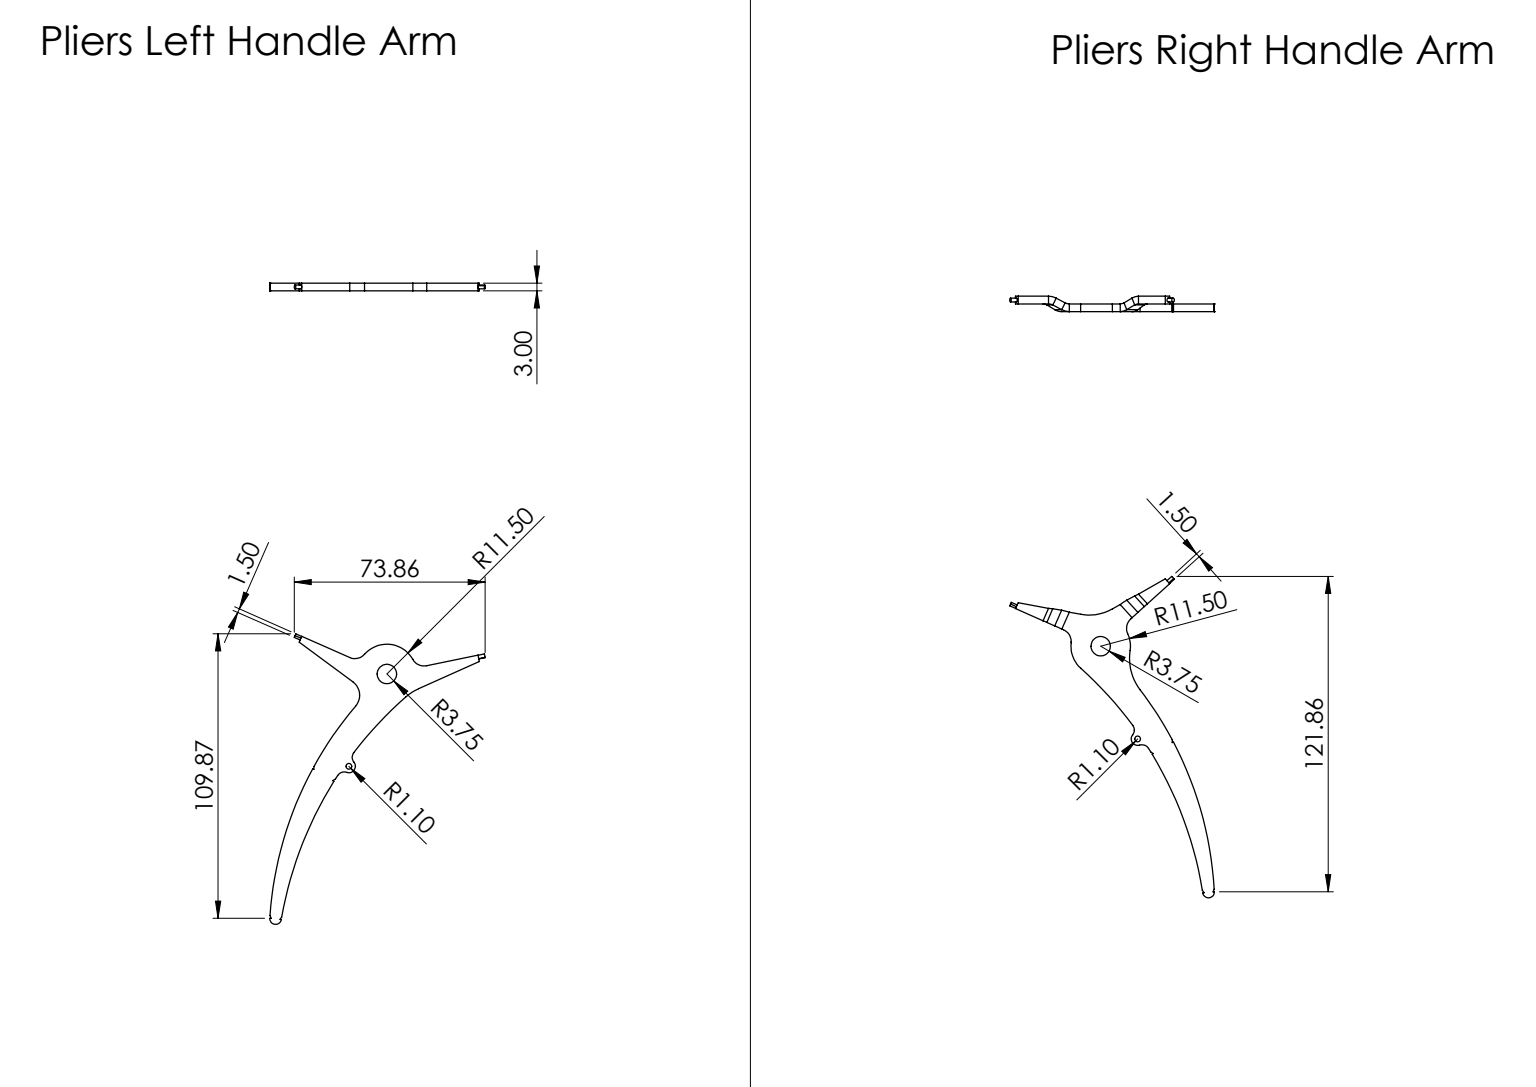
ISO-10303-21;
HEADER;
FILE_DESCRIPTION (('STEP AP214'),
    '1' );
FILE_NAME ('Pliers Left Handle Arm.step',
    '2026-10-09T15:01:35',
    ( '' ),
    ( '' ),
    'SwSTEP 2.0',
    'SolidWorks 2026',
    '' );
FILE_SCHEMA (( 'AUTOMOTIVE_DESIGN' ));
ENDSEC;

DATA;
#3=DIRECTION ( 'NONE',  ( -5.715354789860003484E-18, -9.999836672264337477E-16, 1.000000000000000000 ) ) ;
#4=DIRECTION ( 'NONE',  ( -5.715354789860003484E-18, -9.999836672264337477E-16, 1.000000000000000000 ) ) ;
#12=CARTESIAN_POINT ( 'NONE',  ( 1.714606436958001585E-17, 2.999951001679301835E-15, -3.000000000000000888 ) ) ;
#13=CARTESIAN_POINT ( 'NONE',  ( 37.74350889372263396, 7.597106414893625370, -1.944871132915118705 ) ) ;
#14=CARTESIAN_POINT ( 'NONE',  ( 10.02759472486470926, 5.630039434485818894, -2.999999999999995115 ) ) ;
#21=ORIENTED_EDGE ( 'NONE', *, *, #345, .T. ) ;
#22=ORIENTED_EDGE ( 'NONE', *, *, #4795, .T. ) ;
#27=EDGE_CURVE ( 'NONE', #7442, #6679, #395, .T. ) ;
#42=CYLINDRICAL_SURFACE ( 'NONE', #5055, 2.999999999999999556 ) ;
#44=AXIS2_PLACEMENT_3D ( 'NONE', #1509, #3865, #2736 ) ;
#45=ORIENTED_EDGE ( 'NONE', *, *, #3432, .T. ) ;
#53=CARTESIAN_POINT ( 'NONE',  ( -28.22553731214382111, -35.79092421365019305, -3.595165860846261460E-14 ) ) ;
#55=CARTESIAN_POINT ( 'NONE',  ( -13.19674249314596892, -2.997380612392111843, -3.000000000000003997 ) ) ;
#59=CARTESIAN_POINT ( 'NONE',  ( -14.70408710852078116, -35.66654345889202204, -3.000000000000036415 ) ) ;
#63=DIRECTION ( 'NONE',  ( -5.715354789860003484E-18, -9.999836672264337477E-16, 1.000000000000000000 ) ) ;
#65=ORIENTED_EDGE ( 'NONE', *, *, #2017, .F. ) ;
#74=VERTEX_POINT ( 'NONE', #2232 ) ;
#88=CYLINDRICAL_SURFACE ( 'NONE', #3600, 147.0000000000000284 ) ;
#96=CARTESIAN_POINT ( 'NONE',  ( 30.52077159997833533, 5.488396937353885896, -1.499999999999994893 ) ) ;
#100=DIRECTION ( 'NONE',  ( -0.9999836672264332815, 0.005715354789859956701, 0.000000000000000000 ) ) ;
#112=EDGE_CURVE ( 'NONE', #2053, #3816, #7103, .T. ) ;
#133=FACE_OUTER_BOUND ( 'NONE', #7338, .T. ) ;
#137=ORIENTED_EDGE ( 'NONE', *, *, #2521, .F. ) ;
#142=PLANE ( 'NONE',  #2794 ) ;
#145=CARTESIAN_POINT ( 'NONE',  ( 30.52077159997833533, 5.488396937353885896, -1.499999999999994893 ) ) ;
#155=DIRECTION ( 'NONE',  ( -0.9999836672264332815, 0.005715354789859956701, 0.000000000000000000 ) ) ;
#160=CARTESIAN_POINT ( 'NONE',  ( -28.26642576027046516, -36.90973657692984489, -3.000000000000037748 ) ) ;
#164=AXIS2_PLACEMENT_3D ( 'NONE', #6562, #6008, #5019 ) ;
#168=AXIS2_PLACEMENT_3D ( 'NONE', #4159, #3722, #2491 ) ;
#171=CARTESIAN_POINT ( 'NONE',  ( -16.51707533432788111, -40.85914143033993895, -3.000000000000041744 ) ) ;
#172=ORIENTED_EDGE ( 'NONE', *, *, #3864, .T. ) ;
#173=ORIENTED_EDGE ( 'NONE', *, *, #526, .F. ) ;
#176=CIRCLE ( 'NONE', #6665, 0.7499999999999893419 ) ;
#182=ORIENTED_EDGE ( 'NONE', *, *, #4904, .T. ) ;
#194=DIRECTION ( 'NONE',  ( 9.251858538542970644E-15, 2.775557561562891351E-14, 1.000000000000000000 ) ) ;
#201=DIRECTION ( 'NONE',  ( 0.8552446107963830313, 0.5182245224839744369, 5.231040848230092092E-16 ) ) ;
#211=EDGE_LOOP ( 'NONE', ( #3520, #3050, #137, #3824 ) ) ;
#220=ORIENTED_EDGE ( 'NONE', *, *, #5909, .F. ) ;
#221=DIRECTION ( 'NONE',  ( 0.1200071523045019850, -0.5808948794702039065, -0.8050834878452428622 ) ) ;
#223=DIRECTION ( 'NONE',  ( 0.4039838799357178822, 0.9147661038495488173, -2.999999999999999208E-14 ) ) ;
#225=ORIENTED_EDGE ( 'NONE', *, *, #2234, .T. ) ;
#236=CARTESIAN_POINT ( 'NONE',  ( -19.02987527034469650, -39.22028924617138301, -3.000000000000040412 ) ) ;
#240=CARTESIAN_POINT ( 'NONE',  ( -44.78727511552453677, -94.39397278840091587, -9.464840624037363205E-14 ) ) ;
#244=CARTESIAN_POINT ( 'NONE',  ( -28.68093632328499965, 11.79168739492699913, -1.500000000001999956 ) ) ;
#248=CIRCLE ( 'NONE', #4943, 5.000000000000001776 ) ;
#263=CARTESIAN_POINT ( 'NONE',  ( 12.26605808802378661, -5.710507655519335479, -3.000000000000006661 ) ) ;
#265=VECTOR ( 'NONE', #2707, 999.9999999999998863 ) ;
#270=CARTESIAN_POINT ( 'NONE',  ( -41.31559769795914150, -94.79889909491285493, -3.000000000000095923 ) ) ;
#282=ORIENTED_EDGE ( 'NONE', *, *, #5430, .F. ) ;
#283=ORIENTED_EDGE ( 'NONE', *, *, #2017, .T. ) ;
#286=CIRCLE ( 'NONE', #4504, 147.0000000000000284 ) ;
#293=EDGE_CURVE ( 'NONE', #961, #6756, #1329, .T. ) ;
#297=DIRECTION ( 'NONE',  ( -0.2023178344681509366, 0.9793199139485104787, 9.781476007338054812E-16 ) ) ;
#301=EDGE_LOOP ( 'NONE', ( #225, #3972, #6636, #4802 ) ) ;
#304=EDGE_LOOP ( 'NONE', ( #2533, #3781, #4954, #1609 ) ) ;
#308=DIRECTION ( 'NONE',  ( -5.715354789860003484E-18, -9.999836672264337477E-16, 1.000000000000000000 ) ) ;
#319=ADVANCED_FACE ( 'NONE', ( #794 ), #822, .F. ) ;
#322=CARTESIAN_POINT ( 'NONE',  ( 15.39900769062488806, 3.181283097128406290, -2.999999999999997335 ) ) ;
#329=ORIENTED_EDGE ( 'NONE', *, *, #1529, .F. ) ;
#334=CARTESIAN_POINT ( 'NONE',  ( -33.25476684253261794, 13.81160679460555940, -0.7499999999999977796 ) ) ;
#340=CYLINDRICAL_SURFACE ( 'NONE', #3356, 0.7500000000000000000 ) ;
#341=DIRECTION ( 'NONE',  ( 5.715354789860003484E-18, 9.999836672264337477E-16, -1.000000000000000000 ) ) ;
#342=ORIENTED_EDGE ( 'NONE', *, *, #3838, .T. ) ;
#345=EDGE_CURVE ( 'NONE', #1893, #5033, #4794, .T. ) ;
#347=DIRECTION ( 'NONE',  ( -0.8056443796264689539, 0.5923994712829191434, 5.877852522924718954E-16 ) ) ;
#351=DIRECTION ( 'NONE',  ( -5.715354789860003484E-18, -9.999836672264337477E-16, 1.000000000000000000 ) ) ;
#357=AXIS2_PLACEMENT_3D ( 'NONE', #1661, #431, #1029 ) ;
#364=VERTEX_POINT ( 'NONE', #160 ) ;
#365=EDGE_LOOP ( 'NONE', ( #2898, #4599, #960, #5000 ) ) ;
#366=VECTOR ( 'NONE', #3433, 1000.000000000000000 ) ;
#369=AXIS2_PLACEMENT_3D ( 'NONE', #2221, #569, #5170 ) ;
#384=DIRECTION ( 'NONE',  ( 0.9999836672264332815, -0.005715354789859936752, 0.000000000000000000 ) ) ;
#394=AXIS2_PLACEMENT_3D ( 'NONE', #12, #4824, #4257 ) ;
#395=LINE ( 'NONE', #4507, #6992 ) ;
#398=AXIS2_PLACEMENT_3D ( 'NONE', #5979, #4800, #4664 ) ;
#405=ORIENTED_EDGE ( 'NONE', *, *, #2511, .F. ) ;
#406=ORIENTED_EDGE ( 'NONE', *, *, #5399, .F. ) ;
#411=CARTESIAN_POINT ( 'NONE',  ( -14.70408710852078116, -35.66654345889202204, -3.575000000000001175E-14 ) ) ;
#412=DIRECTION ( 'NONE',  ( -5.715354789860003484E-18, -9.999836672264337477E-16, 1.000000000000000000 ) ) ;
#415=ORIENTED_EDGE ( 'NONE', *, *, #4449, .T. ) ;
#419=EDGE_CURVE ( 'NONE', #7087, #6597, #3623, .T. ) ;
#422=LINE ( 'NONE', #6729, #6529 ) ;
#428=CARTESIAN_POINT ( 'NONE',  ( -28.22553731214382111, -35.79092421365019305, -3.001000000000037193 ) ) ;
#429=EDGE_CURVE ( 'NONE', #3871, #3340, #2130, .T. ) ;
#431=DIRECTION ( 'NONE',  ( 5.715354789860003484E-18, 9.999836672264337477E-16, -1.000000000000000000 ) ) ;
#433=DIRECTION ( 'NONE',  ( -5.715354789860003484E-18, -9.999836672264337477E-16, 1.000000000000000000 ) ) ;
#439=EDGE_CURVE ( 'NONE', #461, #1893, #3908, .T. ) ;
#442=CARTESIAN_POINT ( 'NONE',  ( -20.47590477366745887, -41.48231850745216320, -3.000000000000042633 ) ) ;
#449=ORIENTED_EDGE ( 'NONE', *, *, #4644, .T. ) ;
#461=VERTEX_POINT ( 'NONE', #5084 ) ;
#487=ORIENTED_EDGE ( 'NONE', *, *, #1870, .F. ) ;
#496=CIRCLE ( 'NONE', #1095, 2.500000000000000000 ) ;
#498=DIRECTION ( 'NONE',  ( -0.8795363392562568494, 0.4758317222797389667, 4.707970883985391064E-16 ) ) ;
#499=CARTESIAN_POINT ( 'NONE',  ( -14.70408710852078116, -35.66654345889202204, -3.575000000000001175E-14 ) ) ;
#504=DIRECTION ( 'NONE',  ( 5.715354789860003484E-18, 9.999836672264337477E-16, -1.000000000000000000 ) ) ;
#506=CARTESIAN_POINT ( 'NONE',  ( 1.714606436958001585E-17, 2.999951001679301835E-15, -3.000000000000000888 ) ) ;
#524=DIRECTION ( 'NONE',  ( 5.715354789860003484E-18, 9.999836672264337477E-16, -1.000000000000000000 ) ) ;
#526=EDGE_CURVE ( 'NONE', #6597, #5379, #1712, .T. ) ;
#529=VECTOR ( 'NONE', #1420, 1000.000000000000000 ) ;
#535=DIRECTION ( 'NONE',  ( 0.9999836672264332815, -0.005715354789859183882, 0.000000000000000000 ) ) ;
#537=EDGE_CURVE ( 'NONE', #6624, #4598, #3421, .T. ) ;
#540=CARTESIAN_POINT ( 'NONE',  ( 30.36903322412788242, 6.222886872815382553, -1.499999999999994893 ) ) ;
#543=DIRECTION ( 'NONE',  ( -5.715354789860003484E-18, -9.999836672264337477E-16, 1.000000000000000000 ) ) ;
#554=ORIENTED_EDGE ( 'NONE', *, *, #3471, .F. ) ;
#558=CARTESIAN_POINT ( 'NONE',  ( -33.94153943842304955, 12.25650441806195445, 1.206231629534596424E-14 ) ) ;
#563=ORIENTED_EDGE ( 'NONE', *, *, #5138, .F. ) ;
#564=CARTESIAN_POINT ( 'NONE',  ( 15.39900769062488806, 3.181283097128406290, -2.999999999999997335 ) ) ;
#566=DIRECTION ( 'NONE',  ( 0.9999836672264333925, -0.005715354789860572528, 0.000000000000000000 ) ) ;
#568=DIRECTION ( 'NONE',  ( 5.715354789860003484E-18, 9.999836672264337477E-16, -1.000000000000000000 ) ) ;
#569=DIRECTION ( 'NONE',  ( 0.9793199139485099236, 0.2023178344681530461, 2.079116908177651401E-16 ) ) ;
#577=VERTEX_POINT ( 'NONE', #442 ) ;
#585=CARTESIAN_POINT ( 'NONE',  ( 20.45577244917009097, -23.95683820943715148, -2.383953493077566106E-14 ) ) ;
#587=ORIENTED_EDGE ( 'NONE', *, *, #4643, .F. ) ;
#603=ORIENTED_EDGE ( 'NONE', *, *, #537, .T. ) ;
#613=FACE_OUTER_BOUND ( 'NONE', #5852, .T. ) ;
#615=CARTESIAN_POINT ( 'NONE',  ( -43.04083572346265640, -94.50554989113550164, -9.475000000000005065E-14 ) ) ;
#619=EDGE_CURVE ( 'NONE', #2788, #6597, #2616, .T. ) ;
#620=CARTESIAN_POINT ( 'NONE',  ( -20.47590477366745887, -41.48231850745216320, -4.159866804656187193E-14 ) ) ;
#633=EDGE_CURVE ( 'NONE', #6064, #2053, #1560, .T. ) ;
#646=AXIS2_PLACEMENT_3D ( 'NONE', #1626, #5099, #2826 ) ;
#649=VECTOR ( 'NONE', #1067, 1000.000000000000000 ) ;
#655=FACE_OUTER_BOUND ( 'NONE', #1016, .T. ) ;
#656=AXIS2_PLACEMENT_3D ( 'NONE', #4178, #3567, #4647 ) ;
#664=CARTESIAN_POINT ( 'NONE',  ( 3.749938752099124972, -0.02143258046197201241, -3.000000000000000888 ) ) ;
#668=EDGE_CURVE ( 'NONE', #6756, #3571, #1319, .T. ) ;
#671=DIRECTION ( 'NONE',  ( 0.9147661038495488173, -0.4039838799357178822, 0.000000000000000000 ) ) ;
#680=DIRECTION ( 'NONE',  ( -0.2023178344681547114, 0.9793199139485095905, 8.673617379884032514E-16 ) ) ;
#684=LINE ( 'NONE', #6344, #1217 ) ;
#696=EDGE_LOOP ( 'NONE', ( #3578, #3253, #1799, #5414 ) ) ;
#704=DIRECTION ( 'NONE',  ( -5.715354789860003484E-18, -9.999836672264337477E-16, 1.000000000000000000 ) ) ;
#716=VERTEX_POINT ( 'NONE', #1672 ) ;
#725=FACE_OUTER_BOUND ( 'NONE', #7219, .T. ) ;
#726=ORIENTED_EDGE ( 'NONE', *, *, #2233, .F. ) ;
#730=DIRECTION ( 'NONE',  ( 5.715354789860003484E-18, 9.999836672264337477E-16, -1.000000000000000000 ) ) ;
#741=LINE ( 'NONE', #1289, #2400 ) ;
#746=AXIS2_PLACEMENT_3D ( 'NONE', #4808, #7242, #6749 ) ;
#751=AXIS2_PLACEMENT_3D ( 'NONE', #5959, #3597, #6467 ) ;
#752=DIRECTION ( 'NONE',  ( -0.9147661038495488173, 0.4039838799357178822, 0.000000000000000000 ) ) ;
#759=AXIS2_PLACEMENT_3D ( 'NONE', #3789, #6111, #1904 ) ;
#761=EDGE_CURVE ( 'NONE', #6173, #3671, #7429, .T. ) ;
#776=FACE_OUTER_BOUND ( 'NONE', #2120, .T. ) ;
#781=DIRECTION ( 'NONE',  ( 0.9999836672264332815, -0.005715354789859183882, 0.000000000000000000 ) ) ;
#782=DIRECTION ( 'NONE',  ( 0.9793199139485104787, 0.2023178344681509366, 2.079116908177630447E-16 ) ) ;
#786=EDGE_CURVE ( 'NONE', #5766, #1922, #4465, .T. ) ;
#787=CARTESIAN_POINT ( 'NONE',  ( -10.54744521951312208, -8.271218886098248291, -8.331366185709195643E-15 ) ) ;
#794=FACE_OUTER_BOUND ( 'NONE', #2300, .T. ) ;
#795=CYLINDRICAL_SURFACE ( 'NONE', #5962, 20.00000000000000711 ) ;
#797=UNCERTAINTY_MEASURE_WITH_UNIT (LENGTH_MEASURE( 1.000000000000000082E-05 ), #6381, 'distance_accuracy_value', 'NONE');
#814=ORIENTED_EDGE ( 'NONE', *, *, #429, .F. ) ;
#815=VERTEX_POINT ( 'NONE', #2271 ) ;
#822=CYLINDRICAL_SURFACE ( 'NONE', #4723, 147.0000000000000284 ) ;
#823=VECTOR ( 'NONE', #7264, 1000.000000000000114 ) ;
#836=EDGE_CURVE ( 'NONE', #6064, #5997, #4487, .T. ) ;
#837=EDGE_CURVE ( 'NONE', #716, #1124, #6410, .T. ) ;
#846=PRODUCT ( 'Pliers Left Handle Arm', 'Pliers Left Handle Arm', '', ( #5727 ) ) ;
#847=ADVANCED_FACE ( 'NONE', ( #7018 ), #4192, .T. ) ;
#849=CARTESIAN_POINT ( 'NONE',  ( -16.51707533432788111, -40.85914143033993895, -3.000000000000041744 ) ) ;
#852=ORIENTED_EDGE ( 'NONE', *, *, #5139, .T. ) ;
#853=EDGE_LOOP ( 'NONE', ( #2489, #4961 ) ) ;
#859=VECTOR ( 'NONE', #2007, 1000.000000000000000 ) ;
#860=LINE ( 'NONE', #4298, #4326 ) ;
#868=CARTESIAN_POINT ( 'NONE',  ( -12.80424950550273167, -30.40040925781620373, -3.000000000000031086 ) ) ;
#874=CARTESIAN_POINT ( 'NONE',  ( -28.98392423323637601, 11.10561281704045200, -1.499999999999989564 ) ) ;
#875=CIRCLE ( 'NONE', #4505, 1.100000000000000755 ) ;
#877=ORIENTED_EDGE ( 'NONE', *, *, #633, .F. ) ;
#878=VERTEX_POINT ( 'NONE', #1889 ) ;
#881=FACE_BOUND ( 'NONE', #4518, .T. ) ;
#883=AXIS2_PLACEMENT_3D ( 'NONE', #1572, #1012, #5541 ) ;
#897=CARTESIAN_POINT ( 'NONE',  ( -32.93157973858376408, 14.54341967768581512, 1.435496648130876646E-14 ) ) ;
#908=LINE ( 'NONE', #3797, #4212 ) ;
#910=EDGE_CURVE ( 'NONE', #3970, #2280, #5227, .T. ) ;
#913=FACE_OUTER_BOUND ( 'NONE', #3093, .T. ) ;
#921=DIRECTION ( 'NONE',  ( 0.9793199139485103677, 0.2023178344681514362, 2.079116908177635377E-16 ) ) ;
#922=CARTESIAN_POINT ( 'NONE',  ( 35.25551690214635414, 7.283442040853450372, -2.999999999999993339 ) ) ;
#925=ORIENTED_CLOSED_SHELL ( 'NONE', *, #3017, .F. );
#933=FACE_OUTER_BOUND ( 'NONE', #1417, .T. ) ;
#937=VERTEX_POINT ( 'NONE', #5247 ) ;
#945=EDGE_LOOP ( 'NONE', ( #1825, #3595, #603, #5681 ) ) ;
#952=EDGE_LOOP ( 'NONE', ( #1384, #5365, #5929, #3739 ) ) ;
#960=ORIENTED_EDGE ( 'NONE', *, *, #5662, .F. ) ;
#961=VERTEX_POINT ( 'NONE', #2965 ) ;
#965=DIRECTION ( 'NONE',  ( 0.9999836672264332815, -0.005715354789859975783, 0.000000000000000000 ) ) ;
#967=VECTOR ( 'NONE', #2871, 999.9999999999998863 ) ;
#970=DIRECTION ( 'NONE',  ( -5.715354789860003484E-18, -9.999836672264337477E-16, 1.000000000000000000 ) ) ;
#974=CARTESIAN_POINT ( 'NONE',  ( 20.45577244917009097, -23.95683820943714792, -3.000000000000024869 ) ) ;
#975=LINE ( 'NONE', #7225, #5548 ) ;
#979=EDGE_CURVE ( 'NONE', #3069, #4278, #4033, .T. ) ;
#987=AXIS2_PLACEMENT_3D ( 'NONE', #3584, #3663, #4763 ) ;
#992=DIRECTION ( 'NONE',  ( 5.715354789860003484E-18, 9.999836672264337477E-16, -1.000000000000000000 ) ) ;
#1003=AXIS2_PLACEMENT_3D ( 'NONE', #6627, #2572, #347 ) ;
#1008=AXIS2_PLACEMENT_3D ( 'NONE', #6368, #1212, #704 ) ;
#1012=DIRECTION ( 'NONE',  ( 0.4094857180573137634, -0.9123165276958903336, -9.099612708765444388E-16 ) ) ;
#1016=EDGE_LOOP ( 'NONE', ( #4893, #6389, #4139 ) ) ;
#1017=CARTESIAN_POINT ( 'NONE',  ( -17.04733905648494030, -8.234069079964159599, -8.331366185709195643E-15 ) ) ;
#1020=VECTOR ( 'NONE', #3459, 1000.000000000000000 ) ;
#1022=DIRECTION ( 'NONE',  ( -0.9999836672264332815, 0.005715354789859956701, 0.000000000000000000 ) ) ;
#1023=EDGE_CURVE ( 'NONE', #5766, #716, #1835, .T. ) ;
#1029=DIRECTION ( 'NONE',  ( -0.9999836672264332815, 0.005715354789859956701, 0.000000000000000000 ) ) ;
#1031=EDGE_CURVE ( 'NONE', #2186, #1044, #5088, .T. ) ;
#1036=CARTESIAN_POINT ( 'NONE',  ( -35.54168210215661361, 14.82156649444488394, -1.500000000001999956 ) ) ;
#1037=DIRECTION ( 'NONE',  ( -0.2023178344681514362, 0.9793199139485103677, 9.781476007338052840E-16 ) ) ;
#1040=EDGE_CURVE ( 'NONE', #6066, #5379, #3381, .T. ) ;
#1044=VERTEX_POINT ( 'NONE', #4646 ) ;
#1056=FACE_OUTER_BOUND ( 'NONE', #2951, .T. ) ;
#1058=LINE ( 'NONE', #6298, #1020 ) ;
#1060=DIRECTION ( 'NONE',  ( 0.9999836672264331705, -0.005715354789860001804, 0.000000000000000000 ) ) ;
#1061=ORIENTED_EDGE ( 'NONE', *, *, #2233, .T. ) ;
#1067=DIRECTION ( 'NONE',  ( -5.715354789860003484E-18, -9.999836672264337477E-16, 1.000000000000000000 ) ) ;
#1082=ADVANCED_FACE ( 'NONE', ( #4781 ), #5572, .F. ) ;
#1083=ADVANCED_FACE ( 'NONE', ( #1873 ), #5881, .T. ) ;
#1084=DIRECTION ( 'NONE',  ( 0.3866393274467394559, -0.9222310071080526139, -9.200061635857666883E-16 ) ) ;
#1095=AXIS2_PLACEMENT_3D ( 'NONE', #499, #2173, #4448 ) ;
#1107=ORIENTED_EDGE ( 'NONE', *, *, #4795, .F. ) ;
#1114=VECTOR ( 'NONE', #7078, 1000.000000000000114 ) ;
#1118=EDGE_CURVE ( 'NONE', #3179, #4706, #4817, .T. ) ;
#1119=ORIENTED_EDGE ( 'NONE', *, *, #1682, .F. ) ;
#1121=AXIS2_PLACEMENT_3D ( 'NONE', #4097, #6930, #7411 ) ;
#1122=DIRECTION ( 'NONE',  ( 0.9999836672264331705, -0.005715354789862803382, 0.000000000000000000 ) ) ;
#1124=VERTEX_POINT ( 'NONE', #1348 ) ;
#1134=CIRCLE ( 'NONE', #2685, 0.7499999999999893419 ) ;
#1139=DIRECTION ( 'NONE',  ( -0.4039838799357192700, -0.9147661038495482622, -8.673617379884158732E-16 ) ) ;
#1149=PLANE ( 'NONE',  #3041 ) ;
#1152=CARTESIAN_POINT ( 'NONE',  ( -12.36403222600316276, 10.92614786255227166, -2.999999999999990230 ) ) ;
#1153=EDGE_CURVE ( 'NONE', #7182, #878, #2435, .T. ) ;
#1161=ORIENTED_EDGE ( 'NONE', *, *, #4113, .T. ) ;
#1163=EDGE_LOOP ( 'NONE', ( #5384, #1864 ) ) ;
#1164=SHAPE_DEFINITION_REPRESENTATION ( #1991, #3150 ) ;
#1186=CYLINDRICAL_SURFACE ( 'NONE', #3650, 0.7500000000000000000 ) ;
#1191=ADVANCED_FACE ( 'NONE', ( #5992 ), #142, .F. ) ;
#1207=AXIS2_PLACEMENT_3D ( 'NONE', #974, #6622, #5516 ) ;
#1212=DIRECTION ( 'NONE',  ( -0.9147661038495487063, 0.4039838799357181043, 3.987490689252446030E-16 ) ) ;
#1217=VECTOR ( 'NONE', #4153, 1000.000000000000114 ) ;
#1222=DIRECTION ( 'NONE',  ( 0.1628827478269146978, -0.7884342920379695530, 0.5931615105508275532 ) ) ;
#1223=EDGE_LOOP ( 'NONE', ( #5305, #6325, #1457, #3436 ) ) ;
#1226=PRODUCT_DEFINITION ( 'UNKNOWN', '', #1481, #4879 ) ;
#1230=DIRECTION ( 'NONE',  ( -0.1628827478269146978, 0.7884342920379695530, -0.5931615105508275532 ) ) ;
#1242=VECTOR ( 'NONE', #2762, 1000.000000000000000 ) ;
#1243=ORIENTED_EDGE ( 'NONE', *, *, #2823, .F. ) ;
#1247=DIRECTION ( 'NONE',  ( -5.715354789860003484E-18, -9.999836672264337477E-16, 1.000000000000000000 ) ) ;
#1252=FACE_OUTER_BOUND ( 'NONE', #2627, .T. ) ;
#1256=CIRCLE ( 'NONE', #2447, 0.7499999999999994449 ) ;
#1269=EDGE_CURVE ( 'NONE', #5341, #5266, #1568, .T. ) ;
#1273=VERTEX_POINT ( 'NONE', #7255 ) ;
#1279=FACE_OUTER_BOUND ( 'NONE', #7094, .T. ) ;
#1284=ORIENTED_EDGE ( 'NONE', *, *, #1631, .F. ) ;
#1287=FACE_OUTER_BOUND ( 'NONE', #365, .T. ) ;
#1289=CARTESIAN_POINT ( 'NONE',  ( 12.26605808802378661, -5.710507655519335479, -3.000000000000006661 ) ) ;
#1314=EDGE_CURVE ( 'NONE', #1124, #1044, #1533, .T. ) ;
#1315=DIRECTION ( 'NONE',  ( -0.4039838799357163279, -0.9147661038495494834, -8.673617379884193244E-16 ) ) ;
#1317=CARTESIAN_POINT ( 'NONE',  ( -10.41850315652351533, -32.21925899276746463, -3.227827820482467005E-14 ) ) ;
#1319=LINE ( 'NONE', #4889, #859 ) ;
#1329=LINE ( 'NONE', #270, #3743 ) ;
#1330=AXIS2_PLACEMENT_3D ( 'NONE', #2240, #6279, #1230 ) ;
#1336=DIRECTION ( 'NONE',  ( 0.9999836672264332815, -0.005715354789859876036, 0.000000000000000000 ) ) ;
#1339=VECTOR ( 'NONE', #3728, 1000.000000000000000 ) ;
#1343=EDGE_CURVE ( 'NONE', #7292, #4706, #4493, .T. ) ;
#1346=VECTOR ( 'NONE', #6183, 1000.000000000000000 ) ;
#1348=CARTESIAN_POINT ( 'NONE',  ( -12.20412794045469518, -35.68083184586667045, -3.000000000000036415 ) ) ;
#1349=DIRECTION ( 'NONE',  ( 0.9999836672264333925, -0.005715354789860572528, 0.000000000000000000 ) ) ;
#1352=ORIENTED_EDGE ( 'NONE', *, *, #2823, .T. ) ;
#1356=VECTOR ( 'NONE', #671, 1000.000000000000000 ) ;
#1362=EDGE_CURVE ( 'NONE', #7266, #815, #6525, .T. ) ;
#1380=CARTESIAN_POINT ( 'NONE',  ( -28.26642576027046516, -36.90973657692984489, -3.707068639042112348E-14 ) ) ;
#1384=ORIENTED_EDGE ( 'NONE', *, *, #2180, .T. ) ;
#1385=ORIENTED_EDGE ( 'NONE', *, *, #4441, .T. ) ;
#1386=( NAMED_UNIT ( * ) SI_UNIT ( $, .STERADIAN. ) SOLID_ANGLE_UNIT ( ) );
#1389=CARTESIAN_POINT ( 'NONE',  ( -35.54168210215661361, 14.82156649444488394, -1.500000000001999956 ) ) ;
#1394=PLANE ( 'NONE',  #3148 ) ;
#1407=ORIENTED_EDGE ( 'NONE', *, *, #4065, .F. ) ;
#1409=EDGE_CURVE ( 'NONE', #6990, #1914, #3873, .T. ) ;
#1410=LINE ( 'NONE', #1380, #3507 ) ;
#1417=EDGE_LOOP ( 'NONE', ( #406, #6220, #5612, #7354 ) ) ;
#1420=DIRECTION ( 'NONE',  ( -5.715354789860003484E-18, -9.999836672264337477E-16, 1.000000000000000000 ) ) ;
#1424=FACE_OUTER_BOUND ( 'NONE', #4705, .T. ) ;
#1437=EDGE_CURVE ( 'NONE', #5266, #4706, #6923, .T. ) ;
#1440=ORIENTED_EDGE ( 'NONE', *, *, #6555, .T. ) ;
#1450=ORIENTED_EDGE ( 'NONE', *, *, #7191, .F. ) ;
#1452=VERTEX_POINT ( 'NONE', #4589 ) ;
#1457=ORIENTED_EDGE ( 'NONE', *, *, #1031, .F. ) ;
#1459=ORIENTED_EDGE ( 'NONE', *, *, #6022, .F. ) ;
#1464=AXIS2_PLACEMENT_3D ( 'NONE', #6985, #4168, #1924 ) ;
#1474=CARTESIAN_POINT ( 'NONE',  ( -33.94153943842304955, 12.25650441806195801, -2.999999999999988898 ) ) ;
#1477=CARTESIAN_POINT ( 'NONE',  ( -45.28625779897078729, -94.36209361619114588, -3.000000000000095479 ) ) ;
#1481=PRODUCT_DEFINITION_FORMATION_WITH_SPECIFIED_SOURCE ( 'ANY', '', #846, .NOT_KNOWN. ) ;
#1482=AXIS2_PLACEMENT_3D ( 'NONE', #4523, #5618, #6724 ) ;
#1484=ORIENTED_EDGE ( 'NONE', *, *, #1118, .F. ) ;
#1486=DIRECTION ( 'NONE',  ( -0.9999836672264333925, 0.005715354789860572528, 0.000000000000000000 ) ) ;
#1491=DIRECTION ( 'NONE',  ( -5.715354789860003484E-18, -9.999836672264337477E-16, 1.000000000000000000 ) ) ;
#1493=VERTEX_POINT ( 'NONE', #558 ) ;
#1497=ORIENTED_EDGE ( 'NONE', *, *, #3734, .T. ) ;
#1509=CARTESIAN_POINT ( 'NONE',  ( -20.89962323070193406, -41.21687045383659154, -3.001000000000042078 ) ) ;
#1511=CARTESIAN_POINT ( 'NONE',  ( -35.54168210215661361, 14.82156649444488394, -1.500000000001999956 ) ) ;
#1514=FACE_OUTER_BOUND ( 'NONE', #7021, .T. ) ;
#1529=EDGE_CURVE ( 'NONE', #3340, #1493, #3448, .T. ) ;
#1530=ORIENTED_EDGE ( 'NONE', *, *, #7183, .T. ) ;
#1533=LINE ( 'NONE', #4363, #5219 ) ;
#1552=CARTESIAN_POINT ( 'NONE',  ( 35.76131148831677109, 4.835142255982176174, -2.999999999999995559 ) ) ;
#1553=CIRCLE ( 'NONE', #1207, 20.00000000000000711 ) ;
#1557=CIRCLE ( 'NONE', #2876, 5.000000000000001776 ) ;
#1560=LINE ( 'NONE', #4925, #4116 ) ;
#1562=ORIENTED_EDGE ( 'NONE', *, *, #5909, .T. ) ;
#1568=LINE ( 'NONE', #6759, #3154 ) ;
#1569=EDGE_CURVE ( 'NONE', #3179, #5341, #2207, .T. ) ;
#1572=CARTESIAN_POINT ( 'NONE',  ( 35.76131148831677109, 4.835142255982176174, -2.999999999999995559 ) ) ;
#1578=FACE_OUTER_BOUND ( 'NONE', #5190, .T. ) ;
#1584=ORIENTED_EDGE ( 'NONE', *, *, #4497, .F. ) ;
#1595=AXIS2_PLACEMENT_3D ( 'NONE', #5939, #63, #4163 ) ;
#1600=DIRECTION ( 'NONE',  ( -5.715354789860003484E-18, -9.999836672264337477E-16, 1.000000000000000000 ) ) ;
#1606=DIRECTION ( 'NONE',  ( -5.715354789860003484E-18, -9.999836672264337477E-16, 1.000000000000000000 ) ) ;
#1609=ORIENTED_EDGE ( 'NONE', *, *, #1529, .T. ) ;
#1612=ORIENTED_EDGE ( 'NONE', *, *, #4124, .T. ) ;
#1617=CARTESIAN_POINT ( 'NONE',  ( -32.93157973858376408, 14.54341967768581867, -2.999999999999986677 ) ) ;
#1618=LINE ( 'NONE', #5201, #4369 ) ;
#1621=CARTESIAN_POINT ( 'NONE',  ( -40.82267254781529431, -94.88271315313488685, -9.511447951234663500E-14 ) ) ;
#1623=ORIENTED_EDGE ( 'NONE', *, *, #1963, .F. ) ;
#1626=CARTESIAN_POINT ( 'NONE',  ( 37.86567095459282228, 7.005780695865149177, -1.500000000001998623 ) ) ;
#1631=EDGE_CURVE ( 'NONE', #461, #1922, #3273, .T. ) ;
#1632=ADVANCED_FACE ( 'NONE', ( #133 ), #2502, .F. ) ;
#1649=ORIENTED_EDGE ( 'NONE', *, *, #837, .F. ) ;
#1650=EDGE_CURVE ( 'NONE', #7292, #5643, #1410, .T. ) ;
#1657=ORIENTED_EDGE ( 'NONE', *, *, #4539, .T. ) ;
#1659=DIRECTION ( 'NONE',  ( -0.5182245224839744369, 0.8552446107963831423, 8.522688052730095348E-16 ) ) ;
#1661=CARTESIAN_POINT ( 'NONE',  ( 104.0973215944787711, -119.5240462704291389, -1.189271409856590718E-13 ) ) ;
#1672=CARTESIAN_POINT ( 'NONE',  ( -15.52817266570582611, -38.02681526409561741, -3.000000000000039080 ) ) ;
#1674=ORIENTED_EDGE ( 'NONE', *, *, #5662, .T. ) ;
#1677=AXIS2_PLACEMENT_3D ( 'NONE', #1739, #568, #2134 ) ;
#1679=ORIENTED_EDGE ( 'NONE', *, *, #3432, .F. ) ;
#1682=EDGE_CURVE ( 'NONE', #5997, #3816, #4700, .T. ) ;
#1689=CARTESIAN_POINT ( 'NONE',  ( 94.42889356597736139, -103.2882618349535591, -1.027468802220174526E-13 ) ) ;
#1693=ADVANCED_FACE ( 'NONE', ( #3558 ), #4198, .F. ) ;
#1696=CARTESIAN_POINT ( 'NONE',  ( 30.67250997582947747, 4.753907001892506479, -1.499999999999995559 ) ) ;
#1697=VERTEX_POINT ( 'NONE', #7131 ) ;
#1703=CARTESIAN_POINT ( 'NONE',  ( -20.89962323070193406, -41.21687045383659154, -3.001000000000042078 ) ) ;
#1709=DIRECTION ( 'NONE',  ( -5.715354789860003484E-18, -9.999836672264337477E-16, 1.000000000000000000 ) ) ;
#1712=CIRCLE ( 'NONE', #3509, 140.0000000000000284 ) ;
#1716=ORIENTED_EDGE ( 'NONE', *, *, #6831, .T. ) ;
#1717=ORIENTED_EDGE ( 'NONE', *, *, #1743, .T. ) ;
#1722=CARTESIAN_POINT ( 'NONE',  ( -43.04083572346265640, -94.50554989113550164, -3.000000000000095479 ) ) ;
#1730=VECTOR ( 'NONE', #4636, 1000.000000000000000 ) ;
#1734=AXIS2_PLACEMENT_3D ( 'NONE', #3431, #2261, #3918 ) ;
#1736=LINE ( 'NONE', #2219, #6315 ) ;
#1739=CARTESIAN_POINT ( 'NONE',  ( 104.0973215944787711, -119.5240462704291389, -3.000000000000119904 ) ) ;
#1742=VERTEX_POINT ( 'NONE', #2722 ) ;
#1743=EDGE_CURVE ( 'NONE', #3341, #5578, #2426, .T. ) ;
#1747=DIRECTION ( 'NONE',  ( -0.1628827478269146978, 0.7884342920379695530, -0.5931615105508275532 ) ) ;
#1752=DIRECTION ( 'NONE',  ( -5.715354789860003484E-18, -9.999836672264337477E-16, 1.000000000000000000 ) ) ;
#1772=CARTESIAN_POINT ( 'NONE',  ( -14.70408710852078116, -35.66654345889202204, -3.000000000000036415 ) ) ;
#1773=DIRECTION ( 'NONE',  ( -5.715354789860003484E-18, -9.999836672264337477E-16, 1.000000000000000000 ) ) ;
#1774=EDGE_CURVE ( 'NONE', #3729, #3069, #3776, .T. ) ;
#1775=EDGE_CURVE ( 'NONE', #4598, #1742, #4955, .T. ) ;
#1783=DIRECTION ( 'NONE',  ( 0.9793199139485100346, 0.2023178344681531293, 1.787644449902631965E-16 ) ) ;
#1788=ADVANCED_FACE ( 'NONE', ( #2148 ), #3246, .F. ) ;
#1794=ORIENTED_EDGE ( 'NONE', *, *, #5679, .T. ) ;
#1799=ORIENTED_EDGE ( 'NONE', *, *, #3271, .T. ) ;
#1802=DIRECTION ( 'NONE',  ( 5.715354789860003484E-18, 9.999836672264337477E-16, -1.000000000000000000 ) ) ;
#1807=DIRECTION ( 'NONE',  ( 0.9793199139485101457, 0.2023178344681531016, 2.079116908177651894E-16 ) ) ;
#1814=CIRCLE ( 'NONE', #2647, 0.7500000000000002220 ) ;
#1823=DIRECTION ( 'NONE',  ( 0.9793199139485101457, 0.2023178344681531016, 2.079116908177651894E-16 ) ) ;
#1825=ORIENTED_EDGE ( 'NONE', *, *, #7183, .F. ) ;
#1835=CIRCLE ( 'NONE', #2432, 2.999999999999999556 ) ;
#1840=CYLINDRICAL_SURFACE ( 'NONE', #4375, 147.0000000000000284 ) ;
#1851=ADVANCED_FACE ( 'NONE', ( #881, #4393 ), #4886, .T. ) ;
#1861=DIRECTION ( 'NONE',  ( -5.715354789860003484E-18, -9.999836672264337477E-16, 1.000000000000000000 ) ) ;
#1863=EDGE_LOOP ( 'NONE', ( #1161, #6234, #3613, #4229 ) ) ;
#1864=ORIENTED_EDGE ( 'NONE', *, *, #6450, .T. ) ;
#1870=EDGE_CURVE ( 'NONE', #1742, #6678, #4838, .T. ) ;
#1871=ORIENTED_EDGE ( 'NONE', *, *, #3864, .F. ) ;
#1873=FACE_OUTER_BOUND ( 'NONE', #5304, .T. ) ;
#1889=CARTESIAN_POINT ( 'NONE',  ( 7.283874945971848369, -8.906884184084097100, -8.865108780400335494E-15 ) ) ;
#1892=EDGE_LOOP ( 'NONE', ( #1794, #5333, #4085, #5003 ) ) ;
#1893=VERTEX_POINT ( 'NONE', #3399 ) ;
#1894=DIRECTION ( 'NONE',  ( -5.715354789860003484E-18, -9.999836672264337477E-16, 1.000000000000000000 ) ) ;
#1895=FACE_BOUND ( 'NONE', #2242, .T. ) ;
#1902=DIRECTION ( 'NONE',  ( 0.1200071523045019850, -0.5808948794702039065, -0.8050834878452428622 ) ) ;
#1904=DIRECTION ( 'NONE',  ( -0.4039838799357163279, -0.9147661038495494834, -8.673617379884193244E-16 ) ) ;
#1905=CARTESIAN_POINT ( 'NONE',  ( -40.82267254781529431, -94.88271315313488685, -3.000000000000095923 ) ) ;
#1914=VERTEX_POINT ( 'NONE', #6912 ) ;
#1921=ORIENTED_EDGE ( 'NONE', *, *, #112, .F. ) ;
#1922=VERTEX_POINT ( 'NONE', #2353 ) ;
#1923=AXIS2_PLACEMENT_3D ( 'NONE', #5526, #351, #1336 ) ;
#1924=DIRECTION ( 'NONE',  ( 0.9999836672264331705, -0.005715354789859876036, 0.000000000000000000 ) ) ;
#1925=LINE ( 'NONE', #5300, #7241 ) ;
#1927=ORIENTED_EDGE ( 'NONE', *, *, #4263, .F. ) ;
#1929=ORIENTED_EDGE ( 'NONE', *, *, #6393, .F. ) ;
#1931=AXIS2_PLACEMENT_3D ( 'NONE', #1036, #2750, #7347 ) ;
#1933=DIRECTION ( 'NONE',  ( 0.9793199139485100346, 0.2023178344681531293, 1.804112415015879378E-16 ) ) ;
#1952=AXIS2_PLACEMENT_3D ( 'NONE', #7203, #4349, #6637 ) ;
#1963=EDGE_CURVE ( 'NONE', #3938, #4894, #6275, .T. ) ;
#1964=ORIENTED_EDGE ( 'NONE', *, *, #6706, .T. ) ;
#1974=EDGE_LOOP ( 'NONE', ( #4471, #7057, #3330, #5758 ) ) ;
#1979=FACE_OUTER_BOUND ( 'NONE', #6015, .T. ) ;
#1981=ORIENTED_EDGE ( 'NONE', *, *, #345, .F. ) ;
#1982=EDGE_LOOP ( 'NONE', ( #4442, #7291, #4991, #554 ) ) ;
#1983=ORIENTED_EDGE ( 'NONE', *, *, #5090, .T. ) ;
#1988=EDGE_CURVE ( 'NONE', #6323, #4962, #4721, .T. ) ;
#1991=PRODUCT_DEFINITION_SHAPE ( 'NONE', 'NONE',  #1226 ) ;
#1994=EDGE_CURVE ( 'NONE', #5010, #4166, #4480, .T. ) ;
#2002=ORIENTED_EDGE ( 'NONE', *, *, #4197, .F. ) ;
#2004=DIRECTION ( 'NONE',  ( 5.715354789860003484E-18, 9.999836672264337477E-16, -1.000000000000000000 ) ) ;
#2007=DIRECTION ( 'NONE',  ( -5.715354789860003484E-18, -9.999836672264337477E-16, 1.000000000000000000 ) ) ;
#2017=EDGE_CURVE ( 'NONE', #1697, #7442, #4501, .T. ) ;
#2018=CARTESIAN_POINT ( 'NONE',  ( -28.70619392989860330, -36.67182071578998404, -3.683528784622187242E-14 ) ) ;
#2021=CIRCLE ( 'NONE', #7319, 140.0000000000000284 ) ;
#2022=LINE ( 'NONE', #2103, #823 ) ;
#2024=ORIENTED_EDGE ( 'NONE', *, *, #419, .T. ) ;
#2026=CARTESIAN_POINT ( 'NONE',  ( -28.26642576027046516, -36.90973657692984489, -3.000000000000037748 ) ) ;
#2029=DIRECTION ( 'NONE',  ( -0.2023178344681530183, 0.9793199139485100346, 8.673617379884158732E-16 ) ) ;
#2045=VECTOR ( 'NONE', #5813, 1000.000000000000114 ) ;
#2051=PLANE ( 'NONE',  #4012 ) ;
#2053=VERTEX_POINT ( 'NONE', #4796 ) ;
#2054=ORIENTED_EDGE ( 'NONE', *, *, #761, .F. ) ;
#2061=CARTESIAN_POINT ( 'NONE',  ( -15.80406914246985650, -35.66025656862317561, -3.575000000000001175E-14 ) ) ;
#2066=VECTOR ( 'NONE', #1606, 1000.000000000000000 ) ;
#2070=PLANE ( 'NONE',  #2073 ) ;
#2073=AXIS2_PLACEMENT_3D ( 'NONE', #428, #7230, #6090 ) ;
#2077=CARTESIAN_POINT ( 'NONE',  ( -44.78727511552453677, -94.39397278840091587, -3.000000000000095479 ) ) ;
#2082=DIRECTION ( 'NONE',  ( -0.9979653668924884924, 0.06375834441969779887, 5.805357692931203648E-17 ) ) ;
#2083=VECTOR ( 'NONE', #433, 1000.000000000000000 ) ;
#2094=ORIENTED_EDGE ( 'NONE', *, *, #786, .T. ) ;
#2103=CARTESIAN_POINT ( 'NONE',  ( 37.98783301546301061, 6.414454976836671207, -1.055128867088878541 ) ) ;
#2110=DIRECTION ( 'NONE',  ( -5.715354789860003484E-18, -9.999836672264337477E-16, 1.000000000000000000 ) ) ;
#2120=EDGE_LOOP ( 'NONE', ( #2911, #3182, #6144, #1929 ) ) ;
#2123=DIRECTION ( 'NONE',  ( 1.387778780781445676E-14, 2.775557561562891351E-14, 1.000000000000000000 ) ) ;
#2124=FACE_OUTER_BOUND ( 'NONE', #2862, .T. ) ;
#2125=CARTESIAN_POINT ( 'NONE',  ( -12.75609440306747189, -34.09959597428994726, -3.000000000000035083 ) ) ;
#2129=ADVANCED_FACE ( 'NONE', ( #1514 ), #4417, .F. ) ;
#2130=LINE ( 'NONE', #1617, #7109 ) ;
#2134=DIRECTION ( 'NONE',  ( -0.9999836672264332815, 0.005715354789859956701, 0.000000000000000000 ) ) ;
#2135=DIRECTION ( 'NONE',  ( -5.715354789860003484E-18, -9.999836672264337477E-16, 1.000000000000000000 ) ) ;
#2140=CARTESIAN_POINT ( 'NONE',  ( -20.47590477366745887, -41.48231850745216320, -3.001000000000042522 ) ) ;
#2148=FACE_OUTER_BOUND ( 'NONE', #4292, .T. ) ;
#2149=ADVANCED_BREP_SHAPE_REPRESENTATION ( '', ( #7175, #751 ), #3032 ) ;
#2154=LINE ( 'NONE', #7430, #7216 ) ;
#2157=ORIENTED_EDGE ( 'NONE', *, *, #4559, .F. ) ;
#2163=CYLINDRICAL_SURFACE ( 'NONE', #3535, 2.250000000000031974 ) ;
#2169=LINE ( 'NONE', #5623, #3026 ) ;
#2173=DIRECTION ( 'NONE',  ( -5.715354789860003484E-18, -9.999836672264337477E-16, 1.000000000000000000 ) ) ;
#2176=AXIS2_PLACEMENT_3D ( 'NONE', #615, #2903, #5638 ) ;
#2178=DIRECTION ( 'NONE',  ( -5.715354789860003484E-18, -9.999836672264337477E-16, 1.000000000000000000 ) ) ;
#2180=EDGE_CURVE ( 'NONE', #364, #7163, #3274, .T. ) ;
#2186=VERTEX_POINT ( 'NONE', #3764 ) ;
#2205=AXIS2_PLACEMENT_3D ( 'NONE', #1317, #4711, #4898 ) ;
#2207=LINE ( 'NONE', #4520, #2681 ) ;
#2216=CYLINDRICAL_SURFACE ( 'NONE', #6175, 2.500000000000000000 ) ;
#2219=CARTESIAN_POINT ( 'NONE',  ( 35.25551690214635414, 7.283442040853450372, -2.999999999999993339 ) ) ;
#2221=CARTESIAN_POINT ( 'NONE',  ( 30.52077159997833533, 5.488396937353885896, -1.499999999999994893 ) ) ;
#2224=ADVANCED_FACE ( 'NONE', ( #7339 ), #6194, .F. ) ;
#2230=CARTESIAN_POINT ( 'NONE',  ( -28.22553731214382111, -35.79092421365019305, -3.595165860846261460E-14 ) ) ;
#2231=ORIENTED_EDGE ( 'NONE', *, *, #6450, .F. ) ;
#2232=CARTESIAN_POINT ( 'NONE',  ( 30.67250997583011696, 4.753907001892617501, -1.499999999999995559 ) ) ;
#2233=EDGE_CURVE ( 'NONE', #5807, #6679, #6638, .T. ) ;
#2234=EDGE_CURVE ( 'NONE', #577, #5033, #2824, .T. ) ;
#2239=CARTESIAN_POINT ( 'NONE',  ( -19.02987527034469650, -39.22028924617138301, -3.000000000000040412 ) ) ;
#2240=CARTESIAN_POINT ( 'NONE',  ( 37.86567095459282228, 7.005780695865149177, -1.500000000001998623 ) ) ;
#2242=EDGE_LOOP ( 'NONE', ( #282, #1407 ) ) ;
#2248=DIRECTION ( 'NONE',  ( 0.9222310071080526139, 0.3866393274467394559, 3.919038899579848814E-16 ) ) ;
#2257=CARTESIAN_POINT ( 'NONE',  ( 0.000000000000000000, 0.000000000000000000, 0.000000000000000000 ) ) ;
#2261=DIRECTION ( 'NONE',  ( -0.1676281164441980331, -0.9858503002877112564, -9.867922527762208252E-16 ) ) ;
#2265=LINE ( 'NONE', #1552, #5593 ) ;
#2271=CARTESIAN_POINT ( 'NONE',  ( -28.37794841333321116, 12.47776197281416088, -1.499999999999988010 ) ) ;
#2275=ORIENTED_EDGE ( 'NONE', *, *, #4644, .F. ) ;
#2280=VERTEX_POINT ( 'NONE', #540 ) ;
#2288=CARTESIAN_POINT ( 'NONE',  ( -14.70408710852078116, -35.66654345889202204, -3.000000000000036415 ) ) ;
#2292=CARTESIAN_POINT ( 'NONE',  ( 37.74350889372263396, 7.597106414893625370, -1.944871132915118705 ) ) ;
#2293=LINE ( 'NONE', #4103, #4216 ) ;
#2299=FACE_OUTER_BOUND ( 'NONE', #211, .T. ) ;
#2300=EDGE_LOOP ( 'NONE', ( #5053, #3127, #2094, #1284 ) ) ;
#2312=CARTESIAN_POINT ( 'NONE',  ( -33.94153943842304955, 12.25650441806195801, -2.999999999999988898 ) ) ;
#2313=ORIENTED_EDGE ( 'NONE', *, *, #1682, .T. ) ;
#2315=AXIS2_PLACEMENT_3D ( 'NONE', #59, #1752, #7105 ) ;
#2316=EDGE_LOOP ( 'NONE', ( #5009, #2813, #6458 ) ) ;
#2330=AXIS2_PLACEMENT_3D ( 'NONE', #244, #3064, #6492 ) ;
#2333=DIRECTION ( 'NONE',  ( -0.8474369140690223290, 0.5308961072311347840, 5.260440335992994916E-16 ) ) ;
#2343=ORIENTED_EDGE ( 'NONE', *, *, #4303, .F. ) ;
#2353=CARTESIAN_POINT ( 'NONE',  ( -19.02987527034469650, -39.22028924617138301, -3.932841115884471972E-14 ) ) ;
#2358=ORIENTED_EDGE ( 'NONE', *, *, #5283, .T. ) ;
#2379=FACE_OUTER_BOUND ( 'NONE', #1982, .T. ) ;
#2400=VECTOR ( 'NONE', #1773, 1000.000000000000000 ) ;
#2414=CIRCLE ( 'NONE', #2654, 11.50000000000000178 ) ;
#2422=ORIENTED_EDGE ( 'NONE', *, *, #4441, .F. ) ;
#2426=CIRCLE ( 'NONE', #3880, 2.999999999999999556 ) ;
#2432=AXIS2_PLACEMENT_3D ( 'NONE', #6256, #1802, #566 ) ;
#2435=LINE ( 'NONE', #6469, #3401 ) ;
#2439=CARTESIAN_POINT ( 'NONE',  ( 104.0973215944787711, -119.5240462704291389, -3.000000000000119904 ) ) ;
#2442=VECTOR ( 'NONE', #412, 1000.000000000000000 ) ;
#2447=AXIS2_PLACEMENT_3D ( 'NONE', #6860, #1783, #1222 ) ;
#2454=EDGE_CURVE ( 'NONE', #364, #5643, #4826, .T. ) ;
#2463=CARTESIAN_POINT ( 'NONE',  ( 3.749938752099124972, -0.02143258046197201241, -3.000000000000000888 ) ) ;
#2465=ADVANCED_FACE ( 'NONE', ( #1424 ), #1394, .T. ) ;
#2470=EDGE_LOOP ( 'NONE', ( #5660, #7344, #4658, #3206 ) ) ;
#2471=PLANE ( 'NONE',  #4372 ) ;
#2474=VERTEX_POINT ( 'NONE', #263 ) ;
#2477=ORIENTED_EDGE ( 'NONE', *, *, #293, .F. ) ;
#2480=CARTESIAN_POINT ( 'NONE',  ( 35.25551690214635414, 7.283442040853450372, -2.999999999999993339 ) ) ;
#2483=ORIENTED_EDGE ( 'NONE', *, *, #3799, .T. ) ;
#2489=ORIENTED_EDGE ( 'NONE', *, *, #1994, .T. ) ;
#2491=DIRECTION ( 'NONE',  ( -0.9999836672264332815, 0.005715354789860036498, 0.000000000000000000 ) ) ;
#2500=EDGE_LOOP ( 'NONE', ( #3703, #5611 ) ) ;
#2502=CYLINDRICAL_SURFACE ( 'NONE', #1464, 5.000000000000001776 ) ;
#2503=PLANE ( 'NONE',  #746 ) ;
#2504=EDGE_CURVE ( 'NONE', #3816, #2053, #4360, .T. ) ;
#2511=EDGE_CURVE ( 'NONE', #3571, #4283, #6285, .T. ) ;
#2515=ORIENTED_EDGE ( 'NONE', *, *, #1153, .F. ) ;
#2520=VECTOR ( 'NONE', #5523, 1000.000000000000000 ) ;
#2521=EDGE_CURVE ( 'NONE', #1697, #5807, #3415, .T. ) ;
#2533=ORIENTED_EDGE ( 'NONE', *, *, #4904, .F. ) ;
#2538=CARTESIAN_POINT ( 'NONE',  ( -12.10129460565897475, -12.45149060151658027, -3.000000000000013323 ) ) ;
#2543=ORIENTED_EDGE ( 'NONE', *, *, #4264, .F. ) ;
#2547=AXIS2_PLACEMENT_3D ( 'NONE', #3845, #921, #992 ) ;
#2552=ORIENTED_EDGE ( 'NONE', *, *, #4764, .F. ) ;
#2557=FILL_AREA_STYLE_COLOUR ( '', #4966 ) ;
#2558=VECTOR ( 'NONE', #1037, 999.9999999999998863 ) ;
#2570=DIRECTION ( 'NONE',  ( -5.715354789860003484E-18, -9.999836672264337477E-16, 1.000000000000000000 ) ) ;
#2571=FACE_OUTER_BOUND ( 'NONE', #3843, .T. ) ;
#2572=DIRECTION ( 'NONE',  ( -0.5923994712829191434, -0.8056443796264689539, -8.090169943749487521E-16 ) ) ;
#2585=ORIENTED_EDGE ( 'NONE', *, *, #1569, .F. ) ;
#2588=ORIENTED_EDGE ( 'NONE', *, *, #4065, .T. ) ;
#2616=LINE ( 'NONE', #3290, #4231 ) ;
#2627=EDGE_LOOP ( 'NONE', ( #4810, #5233, #1717, #45 ) ) ;
#2634=ORIENTED_EDGE ( 'NONE', *, *, #2695, .F. ) ;
#2647=AXIS2_PLACEMENT_3D ( 'NONE', #96, #1823, #6427 ) ;
#2654=AXIS2_PLACEMENT_3D ( 'NONE', #506, #6127, #5633 ) ;
#2679=LINE ( 'NONE', #6124, #2520 ) ;
#2680=CARTESIAN_POINT ( 'NONE',  ( -12.80424950550273167, -30.40040925781620729, -3.047309356355731468E-14 ) ) ;
#2681=VECTOR ( 'NONE', #1084, 1000.000000000000000 ) ;
#2685=AXIS2_PLACEMENT_3D ( 'NONE', #5963, #782, #3145 ) ;
#2689=CARTESIAN_POINT ( 'NONE',  ( -45.28625779897078729, -94.36209361619114588, -3.001000000000095813 ) ) ;
#2695=EDGE_CURVE ( 'NONE', #6347, #7087, #1925, .T. ) ;
#2700=ORIENTED_EDGE ( 'NONE', *, *, #1988, .T. ) ;
#2707=DIRECTION ( 'NONE',  ( -0.9793199139485103677, -0.2023178344681514362, -2.079116908177635377E-16 ) ) ;
#2722=CARTESIAN_POINT ( 'NONE',  ( 15.39900769062488806, 3.181283097128403625, 3.269241930315631824E-15 ) ) ;
#2728=VERTEX_POINT ( 'NONE', #5986 ) ;
#2735=DIRECTION ( 'NONE',  ( -0.9999836672264332815, 0.005715354789860036498, 0.000000000000000000 ) ) ;
#2736=DIRECTION ( 'NONE',  ( -0.8474369140690223290, 0.5308961072311346729, 5.260440335992993929E-16 ) ) ;
#2739=CYLINDRICAL_SURFACE ( 'NONE', #7204, 2.500000000000000000 ) ;
#2740=CARTESIAN_POINT ( 'NONE',  ( 1.714606436958001585E-17, 2.999951001679301835E-15, -3.000000000000000888 ) ) ;
#2748=DIRECTION ( 'NONE',  ( 0.9147661038495488173, -0.4039838799357178822, 0.000000000000000000 ) ) ;
#2750=DIRECTION ( 'NONE',  ( -0.9147661038495488173, 0.4039838799357178822, 0.000000000000000000 ) ) ;
#2751=CIRCLE ( 'NONE', #357, 147.0000000000000284 ) ;
#2755=CARTESIAN_POINT ( 'NONE',  ( 35.29520910885068474, 7.091311828723104504, -1.944871132915119150 ) ) ;
#2760=AXIS2_PLACEMENT_3D ( 'NONE', #5519, #341, #1022 ) ;
#2762=DIRECTION ( 'NONE',  ( -5.715354789860003484E-18, -9.999836672264337477E-16, 1.000000000000000000 ) ) ;
#2763=CARTESIAN_POINT ( 'NONE',  ( -43.04083572346265640, -94.50554989113550164, -3.000000000000095479 ) ) ;
#2770=DIRECTION ( 'NONE',  ( 5.715354789860003484E-18, 9.999836672264337477E-16, -1.000000000000000000 ) ) ;
#2779=AXIS2_PLACEMENT_3D ( 'NONE', #3235, #2570, #384 ) ;
#2783=CARTESIAN_POINT ( 'NONE',  ( 35.25551690214635414, 7.283442040853447708, 7.484820869439482625E-15 ) ) ;
#2785=DIRECTION ( 'NONE',  ( 5.715354789860003484E-18, 9.999836672264337477E-16, -1.000000000000000000 ) ) ;
#2787=VECTOR ( 'NONE', #5737, 1000.000000000000114 ) ;
#2788=VERTEX_POINT ( 'NONE', #2538 ) ;
#2794=AXIS2_PLACEMENT_3D ( 'NONE', #4854, #2992, #221 ) ;
#2798=FACE_OUTER_BOUND ( 'NONE', #6354, .T. ) ;
#2809=PLANE ( 'NONE',  #883 ) ;
#2813=ORIENTED_EDGE ( 'NONE', *, *, #7191, .T. ) ;
#2823=EDGE_CURVE ( 'NONE', #1493, #5081, #3024, .T. ) ;
#2824=LINE ( 'NONE', #2140, #5695 ) ;
#2825=ADVANCED_FACE ( 'NONE', ( #6019, #1895, #1279 ), #2471, .T. ) ;
#2826=DIRECTION ( 'NONE',  ( 0.1628827478269146978, -0.7884342920379695530, 0.5931615105508275532 ) ) ;
#2827=CARTESIAN_POINT ( 'NONE',  ( 37.86567095459282228, 7.005780695865149177, -1.500000000001998623 ) ) ;
#2843=CARTESIAN_POINT ( 'NONE',  ( -41.31559769795914150, -94.79889909491285493, -9.503348406515855143E-14 ) ) ;
#2852=CARTESIAN_POINT ( 'NONE',  ( 30.07944552268752503, 5.397223322909749932, -1.499999999999994893 ) ) ;
#2853=LINE ( 'NONE', #4530, #2885 ) ;
#2856=ADVANCED_FACE ( 'NONE', ( #776 ), #2503, .F. ) ;
#2857=DIRECTION ( 'NONE',  ( -0.9147661038495482622, 0.4039838799357193255, 3.987490689252457863E-16 ) ) ;
#2858=FACE_OUTER_BOUND ( 'NONE', #7280, .T. ) ;
#2862=EDGE_LOOP ( 'NONE', ( #220, #5634, #1983, #5635 ) ) ;
#2871=DIRECTION ( 'NONE',  ( 0.8056443796264692869, -0.5923994712829185882, -5.877852522924713037E-16 ) ) ;
#2875=ORIENTED_EDGE ( 'NONE', *, *, #836, .F. ) ;
#2876=AXIS2_PLACEMENT_3D ( 'NONE', #6196, #504, #6782 ) ;
#2882=VECTOR ( 'NONE', #4075, 1000.000000000000227 ) ;
#2884=CARTESIAN_POINT ( 'NONE',  ( 35.25551690214635414, 7.283442040853447708, 7.484820869439482625E-15 ) ) ;
#2885=VECTOR ( 'NONE', #7444, 1000.000000000000227 ) ;
#2897=CARTESIAN_POINT ( 'NONE',  ( -28.26642576027046516, -36.90973657692984489, -3.707068639042112348E-14 ) ) ;
#2898=ORIENTED_EDGE ( 'NONE', *, *, #5554, .T. ) ;
#2903=DIRECTION ( 'NONE',  ( -5.715354789860003484E-18, -9.999836672264337477E-16, 1.000000000000000000 ) ) ;
#2904=CARTESIAN_POINT ( 'NONE',  ( -45.21893524706405287, -93.36435596057614816, -3.000000000000094591 ) ) ;
#2908=AXIS2_PLACEMENT_3D ( 'NONE', #7069, #7097, #1315 ) ;
#2910=CARTESIAN_POINT ( 'NONE',  ( -12.36403222600316276, 10.92614786255226811, 1.085530457744840442E-14 ) ) ;
#2911=ORIENTED_EDGE ( 'NONE', *, *, #293, .T. ) ;
#2913=ORIENTED_EDGE ( 'NONE', *, *, #3831, .F. ) ;
#2914=AXIS2_PLACEMENT_3D ( 'NONE', #6109, #4965, #965 ) ;
#2916=DIRECTION ( 'NONE',  ( -5.715354789860003484E-18, -9.999836672264337477E-16, 1.000000000000000000 ) ) ;
#2926=CIRCLE ( 'NONE', #4982, 3.750000000000000444 ) ;
#2937=CIRCLE ( 'NONE', #3768, 2.500000000000000000 ) ;
#2944=ORIENTED_EDGE ( 'NONE', *, *, #6642, .F. ) ;
#2947=CARTESIAN_POINT ( 'NONE',  ( 35.76131148831677109, 4.835142255982173509, 5.039451867604972471E-15 ) ) ;
#2950=DIRECTION ( 'NONE',  ( 5.715354789860003484E-18, 9.999836672264337477E-16, -1.000000000000000000 ) ) ;
#2951=EDGE_LOOP ( 'NONE', ( #3730, #4935, #1716, #2157 ) ) ;
#2952=ORIENTED_EDGE ( 'NONE', *, *, #5378, .F. ) ;
#2965=CARTESIAN_POINT ( 'NONE',  ( -41.31559769795914150, -94.79889909491285493, -3.000000000000095923 ) ) ;
#2968=DIRECTION ( 'NONE',  ( -0.9147661038495489283, 0.4039838799357176602, 3.987490689252441100E-16 ) ) ;
#2975=DIRECTION ( 'NONE',  ( 0.9147661038495488173, -0.4039838799357178822, 0.000000000000000000 ) ) ;
#2984=ORIENTED_EDGE ( 'NONE', *, *, #4687, .T. ) ;
#2992=DIRECTION ( 'NONE',  ( 0.9793199139485100346, 0.2023178344681531293, 1.804112415015879378E-16 ) ) ;
#2996=EDGE_CURVE ( 'NONE', #4883, #6624, #6206, .T. ) ;
#3008=CARTESIAN_POINT ( 'NONE',  ( -35.54168210215661361, 14.82156649444488394, -1.500000000001999956 ) ) ;
#3012=DIRECTION ( 'NONE',  ( 0.9999836672264332815, -0.005715354789859975783, 0.000000000000000000 ) ) ;
#3016=DIRECTION ( 'NONE',  ( 0.9999836672264331705, -0.005715354789859876036, 0.000000000000000000 ) ) ;
#3017=CLOSED_SHELL ( 'NONE', ( #1082, #6699, #1693 ) ) ;
#3019=ORIENTED_EDGE ( 'NONE', *, *, #1023, .F. ) ;
#3024=LINE ( 'NONE', #6433, #5704 ) ;
#3026=VECTOR ( 'NONE', #4409, 999.9999999999998863 ) ;
#3032=( GEOMETRIC_REPRESENTATION_CONTEXT ( 3 ) GLOBAL_UNCERTAINTY_ASSIGNED_CONTEXT ( ( #5400 ) ) GLOBAL_UNIT_ASSIGNED_CONTEXT ( ( #4209, #7035, #1386 ) ) REPRESENTATION_CONTEXT ( 'NONE', 'WORKASPACE' ) );
#3038=FACE_OUTER_BOUND ( 'NONE', #301, .T. ) ;
#3041=AXIS2_PLACEMENT_3D ( 'NONE', #7340, #1659, #6857 ) ;
#3044=VECTOR ( 'NONE', #201, 1000.000000000000000 ) ;
#3045=CIRCLE ( 'NONE', #5106, 6.500000000000001776 ) ;
#3050=ORIENTED_EDGE ( 'NONE', *, *, #5872, .T. ) ;
#3060=FACE_OUTER_BOUND ( 'NONE', #5291, .T. ) ;
#3064=DIRECTION ( 'NONE',  ( -0.9147661038495488173, 0.4039838799357178822, 1.577721810442023611E-30 ) ) ;
#3069=VERTEX_POINT ( 'NONE', #2947 ) ;
#3075=EDGE_LOOP ( 'NONE', ( #6136, #4863, #6461, #4194 ) ) ;
#3076=( NAMED_UNIT ( * ) PLANE_ANGLE_UNIT ( ) SI_UNIT ( $, .RADIAN. ) );
#3085=CARTESIAN_POINT ( 'NONE',  ( 20.45577244917009097, -23.95683820943714792, -3.000000000000024869 ) ) ;
#3093=EDGE_LOOP ( 'NONE', ( #1243, #329, #6377, #2483 ) ) ;
#3100=VERTEX_POINT ( 'NONE', #14 ) ;
#3112=CIRCLE ( 'NONE', #4207, 3.750000000000000444 ) ;
#3120=CIRCLE ( 'NONE', #7337, 11.50000000000000178 ) ;
#3127=ORIENTED_EDGE ( 'NONE', *, *, #4764, .T. ) ;
#3145=DIRECTION ( 'NONE',  ( -0.2023178344681530183, 0.9793199139485100346, 8.673617379884158732E-16 ) ) ;
#3148=AXIS2_PLACEMENT_3D ( 'NONE', #6803, #5038, #5076 ) ;
#3150=SHAPE_REPRESENTATION ( 'Pliers Left Handle Arm', ( #751 ), #3032 ) ;
#3154=VECTOR ( 'NONE', #6692, 1000.000000000000000 ) ;
#3179=VERTEX_POINT ( 'NONE', #2904 ) ;
#3182=ORIENTED_EDGE ( 'NONE', *, *, #668, .T. ) ;
#3206=ORIENTED_EDGE ( 'NONE', *, *, #5925, .T. ) ;
#3215=ORIENTED_EDGE ( 'NONE', *, *, #4072, .T. ) ;
#3229=DIRECTION ( 'NONE',  ( 0.9999836672264332815, -0.005715354789859975783, 0.000000000000000000 ) ) ;
#3235=CARTESIAN_POINT ( 'NONE',  ( -14.70408710852078116, -35.66654345889202204, -3.000000000000036415 ) ) ;
#3246=PLANE ( 'NONE',  #6166 ) ;
#3253=ORIENTED_EDGE ( 'NONE', *, *, #4124, .F. ) ;
#3257=LINE ( 'NONE', #2125, #6078 ) ;
#3267=DIRECTION ( 'NONE',  ( -5.715354789860003484E-18, -9.999836672264337477E-16, 1.000000000000000000 ) ) ;
#3271=EDGE_CURVE ( 'NONE', #2474, #4883, #4118, .T. ) ;
#3273=CIRCLE ( 'NONE', #4616, 147.0000000000000284 ) ;
#3274=LINE ( 'NONE', #2026, #5211 ) ;
#3278=VECTOR ( 'NONE', #7310, 1000.000000000000114 ) ;
#3290=CARTESIAN_POINT ( 'NONE',  ( -12.10129460565897475, -12.45149060151658027, -3.000000000000013323 ) ) ;
#3291=CARTESIAN_POINT ( 'NONE',  ( 35.76131148831677109, 4.835142255982176174, -2.999999999999995559 ) ) ;
#3293=EDGE_CURVE ( 'NONE', #815, #7266, #6073, .T. ) ;
#3295=EDGE_LOOP ( 'NONE', ( #6436, #6920, #5073 ) ) ;
#3305=CARTESIAN_POINT ( 'NONE',  ( -19.94212619460463287, -40.63668738334721553, -4.075000000000002200E-14 ) ) ;
#3313=DIRECTION ( 'NONE',  ( 0.9999836672264332815, -0.005715354789860036498, 0.000000000000000000 ) ) ;
#3315=ADVANCED_FACE ( 'NONE', ( #913 ), #5596, .T. ) ;
#3330=ORIENTED_EDGE ( 'NONE', *, *, #1118, .T. ) ;
#3332=DIRECTION ( 'NONE',  ( -5.715354789860003484E-18, -9.999836672264337477E-16, 1.000000000000000000 ) ) ;
#3337=CARTESIAN_POINT ( 'NONE',  ( -41.31559769795914150, -94.79889909491285493, -3.001000000000096257 ) ) ;
#3340=VERTEX_POINT ( 'NONE', #1474 ) ;
#3341=VERTEX_POINT ( 'NONE', #4453 ) ;
#3344=DIRECTION ( 'NONE',  ( -5.715354789860003484E-18, -9.999836672264337477E-16, 1.000000000000000000 ) ) ;
#3355=DIRECTION ( 'NONE',  ( 0.9999836672264331705, -0.005715354789860001804, 0.000000000000000000 ) ) ;
#3356=AXIS2_PLACEMENT_3D ( 'NONE', #1511, #6703, #3796 ) ;
#3373=AXIS2_PLACEMENT_3D ( 'NONE', #585, #2950, #5265 ) ;
#3379=ADVANCED_FACE ( 'NONE', ( #3802 ), #2070, .F. ) ;
#3380=DIRECTION ( 'NONE',  ( 0.9999836672264332815, -0.005715354789859183882, 0.000000000000000000 ) ) ;
#3381=LINE ( 'NONE', #6400, #4728 ) ;
#3383=CARTESIAN_POINT ( 'NONE',  ( -14.70408710852078116, -35.66654345889202204, -3.000000000000036415 ) ) ;
#3392=DIRECTION ( 'NONE',  ( -5.715354789860003484E-18, -9.999836672264337477E-16, 1.000000000000000000 ) ) ;
#3395=AXIS2_PLACEMENT_3D ( 'NONE', #7381, #2857, #5777 ) ;
#3399=CARTESIAN_POINT ( 'NONE',  ( -20.89962323070193406, -41.21687045383659154, -4.133564602976221858E-14 ) ) ;
#3401=VECTOR ( 'NONE', #6029, 1000.000000000000000 ) ;
#3409=VERTEX_POINT ( 'NONE', #4305 ) ;
#3411=CIRCLE ( 'NONE', #168, 6.500000000000001776 ) ;
#3415=LINE ( 'NONE', #6838, #1356 ) ;
#3421=LINE ( 'NONE', #564, #265 ) ;
#3431=CARTESIAN_POINT ( 'NONE',  ( -40.82267254781529431, -94.88271315313488685, -3.001000000000096257 ) ) ;
#3432=EDGE_CURVE ( 'NONE', #5578, #7025, #6123, .T. ) ;
#3433=DIRECTION ( 'NONE',  ( -5.715354789860003484E-18, -9.999836672264337477E-16, 1.000000000000000000 ) ) ;
#3435=DIRECTION ( 'NONE',  ( 0.9793199139485099236, 0.2023178344681530461, 2.079116908177651401E-16 ) ) ;
#3436=ORIENTED_EDGE ( 'NONE', *, *, #6628, .F. ) ;
#3442=CARTESIAN_POINT ( 'NONE',  ( -8.617355793880991044, 7.615193964809154004, -2.999999999999993339 ) ) ;
#3448=LINE ( 'NONE', #5844, #1730 ) ;
#3449=EDGE_LOOP ( 'NONE', ( #6815, #5042, #4423, #1484 ) ) ;
#3458=DIRECTION ( 'NONE',  ( -0.2023178344681514362, 0.9793199139485103677, 9.781476007338052840E-16 ) ) ;
#3459=DIRECTION ( 'NONE',  ( -5.715354789860003484E-18, -9.999836672264337477E-16, 1.000000000000000000 ) ) ;
#3460=DIRECTION ( 'NONE',  ( -5.715354789860003484E-18, -9.999836672264337477E-16, 1.000000000000000000 ) ) ;
#3465=CYLINDRICAL_SURFACE ( 'NONE', #6309, 11.50000000000000178 ) ;
#3468=CARTESIAN_POINT ( 'NONE',  ( -17.04733905648494030, -8.234069079964157822, -3.000000000000009326 ) ) ;
#3471=EDGE_CURVE ( 'NONE', #3938, #4842, #3878, .T. ) ;
#3489=CARTESIAN_POINT ( 'NONE',  ( -35.54168210215660650, 14.82156649444490348, -0.7500000000019999558 ) ) ;
#3492=DIRECTION ( 'NONE',  ( -5.715354789860003484E-18, -9.999836672264337477E-16, 1.000000000000000000 ) ) ;
#3493=PLANE ( 'NONE',  #1008 ) ;
#3495=LINE ( 'NONE', #1696, #2045 ) ;
#3500=CLOSED_SHELL ( 'NONE', ( #5646, #4777, #1191 ) ) ;
#3507=VECTOR ( 'NONE', #6460, 1000.000000000000000 ) ;
#3509=AXIS2_PLACEMENT_3D ( 'NONE', #1689, #4561, #3984 ) ;
#3520=ORIENTED_EDGE ( 'NONE', *, *, #27, .T. ) ;
#3521=EDGE_LOOP ( 'NONE', ( #4696, #1061, #6283, #65 ) ) ;
#3528=ADVANCED_FACE ( 'NONE', ( #6308 ), #7418, .F. ) ;
#3529=AXIS2_PLACEMENT_3D ( 'NONE', #6945, #1709, #5223 ) ;
#3531=EDGE_LOOP ( 'NONE', ( #7162, #2515, #172, #1612 ) ) ;
#3532=CIRCLE ( 'NONE', #6773, 5.000000000000001776 ) ;
#3535=AXIS2_PLACEMENT_3D ( 'NONE', #2763, #6286, #5686 ) ;
#3545=LINE ( 'NONE', #1703, #366 ) ;
#3554=ORIENTED_EDGE ( 'NONE', *, *, #979, .T. ) ;
#3557=ADVANCED_FACE ( 'NONE', ( #5664 ), #1149, .F. ) ;
#3558=FACE_OUTER_BOUND ( 'NONE', #5591, .T. ) ;
#3565=ADVANCED_FACE ( 'NONE', ( #2858 ), #3465, .T. ) ;
#3566=DIRECTION ( 'NONE',  ( -5.715354789860003484E-18, -9.999836672264337477E-16, 1.000000000000000000 ) ) ;
#3567=DIRECTION ( 'NONE',  ( -5.715354789860003484E-18, -9.999836672264337477E-16, 1.000000000000000000 ) ) ;
#3571=VERTEX_POINT ( 'NONE', #6903 ) ;
#3578=ORIENTED_EDGE ( 'NONE', *, *, #1774, .F. ) ;
#3579=CARTESIAN_POINT ( 'NONE',  ( -20.89962323070193406, -41.21687045383659154, -4.133564602976221858E-14 ) ) ;
#3580=DIRECTION ( 'NONE',  ( -5.715354789860003484E-18, -9.999836672264337477E-16, 1.000000000000000000 ) ) ;
#3584=CARTESIAN_POINT ( 'NONE',  ( 94.42889356597736139, -103.2882618349535591, -3.000000000000103917 ) ) ;
#3585=FACE_BOUND ( 'NONE', #1163, .T. ) ;
#3595=ORIENTED_EDGE ( 'NONE', *, *, #5925, .F. ) ;
#3596=CIRCLE ( 'NONE', #5543, 0.7499999999999893419 ) ;
#3597=DIRECTION ( 'NONE',  ( 0.000000000000000000, 0.000000000000000000, 1.000000000000000000 ) ) ;
#3600=AXIS2_PLACEMENT_3D ( 'NONE', #6940, #543, #4108 ) ;
#3602=CARTESIAN_POINT ( 'NONE',  ( -10.41850315652351533, -32.21925899276746463, -3.000000000000032863 ) ) ;
#3606=CONICAL_SURFACE ( 'NONE', #369, 0.7500000000000002220, 1.029744258676651425 ) ;
#3611=CIRCLE ( 'NONE', #4595, 2.999999999999999556 ) ;
#3613=ORIENTED_EDGE ( 'NONE', *, *, #3987, .T. ) ;
#3623=CIRCLE ( 'NONE', #3995, 6.500000000000001776 ) ;
#3629=DIRECTION ( 'NONE',  ( -5.715354789860004255E-18, -9.999836672264337477E-16, 1.000000000000000000 ) ) ;
#3636=VECTOR ( 'NONE', #6753, 1000.000000000000000 ) ;
#3645=DIRECTION ( 'NONE',  ( -5.715354789860003484E-18, -9.999836672264337477E-16, 1.000000000000000000 ) ) ;
#3648=FACE_OUTER_BOUND ( 'NONE', #4327, .T. ) ;
#3650=AXIS2_PLACEMENT_3D ( 'NONE', #3008, #2975, #4110 ) ;
#3660=FACE_OUTER_BOUND ( 'NONE', #3531, .T. ) ;
#3663=DIRECTION ( 'NONE',  ( -5.715354789860003484E-18, -9.999836672264337477E-16, 1.000000000000000000 ) ) ;
#3671=VERTEX_POINT ( 'NONE', #4790 ) ;
#3676=CYLINDRICAL_SURFACE ( 'NONE', #4977, 2.999999999999999556 ) ;
#3685=ORIENTED_EDGE ( 'NONE', *, *, #1775, .F. ) ;
#3697=ORIENTED_EDGE ( 'NONE', *, *, #2454, .T. ) ;
#3699=CARTESIAN_POINT ( 'NONE',  ( 104.0973215944787711, -119.5240462704291389, -1.189271409856590718E-13 ) ) ;
#3700=DIRECTION ( 'NONE',  ( 0.9999836672264332815, -0.005715354789860001804, 0.000000000000000000 ) ) ;
#3703=ORIENTED_EDGE ( 'NONE', *, *, #5147, .F. ) ;
#3718=CIRCLE ( 'NONE', #2760, 147.0000000000000284 ) ;
#3722=DIRECTION ( 'NONE',  ( 5.715354789860003484E-18, 9.999836672264337477E-16, -1.000000000000000000 ) ) ;
#3728=DIRECTION ( 'NONE',  ( -0.8174211450113090249, -0.5760405121937176576, -5.807029557109402914E-16 ) ) ;
#3729=VERTEX_POINT ( 'NONE', #4716 ) ;
#3730=ORIENTED_EDGE ( 'NONE', *, *, #1314, .F. ) ;
#3734=EDGE_CURVE ( 'NONE', #7442, #1697, #6480, .T. ) ;
#3739=ORIENTED_EDGE ( 'NONE', *, *, #2454, .F. ) ;
#3743=VECTOR ( 'NONE', #6005, 1000.000000000000114 ) ;
#3749=AXIS2_PLACEMENT_3D ( 'NONE', #6780, #2178, #3313 ) ;
#3750=AXIS2_PLACEMENT_3D ( 'NONE', #5913, #1933, #1902 ) ;
#3751=ORIENTED_EDGE ( 'NONE', *, *, #4497, .T. ) ;
#3764=CARTESIAN_POINT ( 'NONE',  ( -15.52817266570582611, -38.02681526409561741, -3.811494319675517002E-14 ) ) ;
#3768=AXIS2_PLACEMENT_3D ( 'NONE', #7070, #3492, #781 ) ;
#3776=LINE ( 'NONE', #5027, #3278 ) ;
#3781=ORIENTED_EDGE ( 'NONE', *, *, #5487, .F. ) ;
#3789=CARTESIAN_POINT ( 'NONE',  ( -28.68093632328457332, 11.79168739492758711, -1.499999999999988676 ) ) ;
#3796=DIRECTION ( 'NONE',  ( -9.251858538542970644E-15, -2.775557561562891351E-14, -1.000000000000000000 ) ) ;
#3797=CARTESIAN_POINT ( 'NONE',  ( -19.94212619460463287, -40.63668738334721553, -3.001000000000041634 ) ) ;
#3799=EDGE_CURVE ( 'NONE', #5544, #5081, #860, .T. ) ;
#3802=FACE_OUTER_BOUND ( 'NONE', #7058, .T. ) ;
#3804=DIRECTION ( 'NONE',  ( -0.9999836672264332815, 0.005715354789860036498, 0.000000000000000000 ) ) ;
#3816=VERTEX_POINT ( 'NONE', #2061 ) ;
#3824=ORIENTED_EDGE ( 'NONE', *, *, #3734, .F. ) ;
#3831=EDGE_CURVE ( 'NONE', #7163, #3179, #2021, .T. ) ;
#3833=ORIENTED_EDGE ( 'NONE', *, *, #633, .T. ) ;
#3834=AXIS2_PLACEMENT_3D ( 'NONE', #6851, #6732, #498 ) ;
#3838=EDGE_CURVE ( 'NONE', #4842, #2728, #2022, .T. ) ;
#3843=EDGE_LOOP ( 'NONE', ( #5160, #173, #7398, #3751 ) ) ;
#3845=CARTESIAN_POINT ( 'NONE',  ( 35.25551690214635414, 7.283442040853450372, -2.999999999999993339 ) ) ;
#3849=DIRECTION ( 'NONE',  ( -5.715354789860003484E-18, -9.999836672264337477E-16, 1.000000000000000000 ) ) ;
#3853=ORIENTED_EDGE ( 'NONE', *, *, #4264, .T. ) ;
#3857=AXIS2_PLACEMENT_3D ( 'NONE', #6421, #4659, #5180 ) ;
#3859=FACE_OUTER_BOUND ( 'NONE', #3449, .T. ) ;
#3864=EDGE_CURVE ( 'NONE', #7182, #2474, #1553, .T. ) ;
#3865=DIRECTION ( 'NONE',  ( -0.5308961072311346729, -0.8474369140690223290, -8.504573326831746910E-16 ) ) ;
#3871=VERTEX_POINT ( 'NONE', #5549 ) ;
#3873=CIRCLE ( 'NONE', #5705, 2.250000000000031974 ) ;
#3874=ADVANCED_FACE ( 'NONE', ( #5588 ), #340, .T. ) ;
#3878=CIRCLE ( 'NONE', #646, 0.7499999999999994449 ) ;
#3880=AXIS2_PLACEMENT_3D ( 'NONE', #4993, #2004, #1486 ) ;
#3886=ORIENTED_EDGE ( 'NONE', *, *, #4532, .T. ) ;
#3903=CARTESIAN_POINT ( 'NONE',  ( -45.28625779897078729, -94.36209361619114588, -9.461937945190903839E-14 ) ) ;
#3908=LINE ( 'NONE', #3305, #1346 ) ;
#3911=PLANE ( 'NONE',  #3834 ) ;
#3914=ORIENTED_EDGE ( 'NONE', *, *, #6706, .F. ) ;
#3916=ORIENTED_EDGE ( 'NONE', *, *, #7022, .F. ) ;
#3918=DIRECTION ( 'NONE',  ( -0.9858503002877112564, 0.1676281164441980331, 1.619908943762944784E-16 ) ) ;
#3921=LINE ( 'NONE', #5144, #649 ) ;
#3932=EDGE_CURVE ( 'NONE', #5578, #7182, #4082, .T. ) ;
#3938=VERTEX_POINT ( 'NONE', #2292 ) ;
#3940=CYLINDRICAL_SURFACE ( 'NONE', #1482, 3.750000000000000444 ) ;
#3952=CARTESIAN_POINT ( 'NONE',  ( 104.0973215944787711, -119.5240462704291389, -3.000000000000119904 ) ) ;
#3959=AXIS2_PLACEMENT_3D ( 'NONE', #145, #1807, #680 ) ;
#3965=VECTOR ( 'NONE', #6735, 1000.000000000000000 ) ;
#3970=VERTEX_POINT ( 'NONE', #2852 ) ;
#3972=ORIENTED_EDGE ( 'NONE', *, *, #4687, .F. ) ;
#3984=DIRECTION ( 'NONE',  ( 0.9999836672264332815, -0.005715354789859975783, 0.000000000000000000 ) ) ;
#3987=EDGE_CURVE ( 'NONE', #4283, #4962, #6260, .T. ) ;
#3995=AXIS2_PLACEMENT_3D ( 'NONE', #1017, #2770, #2735 ) ;
#3999=LINE ( 'NONE', #6310, #6731 ) ;
#4001=CARTESIAN_POINT ( 'NONE',  ( 30.52077159997833533, 5.488396937353885896, -1.499999999999994893 ) ) ;
#4012=AXIS2_PLACEMENT_3D ( 'NONE', #1389, #7071, #223 ) ;
#4017=ADVANCED_FACE ( 'NONE', ( #4565 ), #3911, .F. ) ;
#4031=ORIENTED_EDGE ( 'NONE', *, *, #1343, .T. ) ;
#4033=LINE ( 'NONE', #2884, #4368 ) ;
#4039=ADVANCED_FACE ( 'NONE', ( #6300 ), #2739, .T. ) ;
#4048=SURFACE_SIDE_STYLE ('',( #5181 ) ) ;
#4065=EDGE_CURVE ( 'NONE', #7056, #1273, #3112, .T. ) ;
#4069=CARTESIAN_POINT ( 'NONE',  ( -12.75609440306747189, -34.09959597428994726, -3.417194463855666027E-14 ) ) ;
#4072=EDGE_CURVE ( 'NONE', #4319, #3871, #6471, .T. ) ;
#4075=DIRECTION ( 'NONE',  ( 0.03652191451860400950, 0.9993328523369456873, 9.995252661588299226E-16 ) ) ;
#4078=SURFACE_STYLE_USAGE ( .BOTH. , #4048 ) ;
#4082=CIRCLE ( 'NONE', #1677, 147.0000000000000284 ) ;
#4085=ORIENTED_EDGE ( 'NONE', *, *, #439, .T. ) ;
#4090=DIRECTION ( 'NONE',  ( -0.5941197849118597940, -0.8043765792067080200, -8.077590468646243185E-16 ) ) ;
#4094=AXIS2_PLACEMENT_3D ( 'NONE', #5288, #4612, #4571 ) ;
#4097=CARTESIAN_POINT ( 'NONE',  ( -14.70408710852078116, -35.66654345889202204, -3.575000000000001175E-14 ) ) ;
#4098=CIRCLE ( 'NONE', #3373, 20.00000000000000711 ) ;
#4103=CARTESIAN_POINT ( 'NONE',  ( -45.28625779897078729, -94.36209361619114588, -9.461937945190903839E-14 ) ) ;
#4105=ADVANCED_FACE ( 'NONE', ( #1252 ), #42, .F. ) ;
#4108=DIRECTION ( 'NONE',  ( 0.9999836672264332815, -0.005715354789859956701, 0.000000000000000000 ) ) ;
#4110=DIRECTION ( 'NONE',  ( -9.251858538542970644E-15, -2.775557561562891351E-14, -1.000000000000000000 ) ) ;
#4113=EDGE_CURVE ( 'NONE', #1914, #961, #4180, .T. ) ;
#4116=VECTOR ( 'NONE', #3849, 1000.000000000000000 ) ;
#4118=LINE ( 'NONE', #4189, #4622 ) ;
#4124=EDGE_CURVE ( 'NONE', #2474, #3729, #741, .T. ) ;
#4125=EDGE_CURVE ( 'NONE', #74, #2280, #6145, .T. ) ;
#4129=VECTOR ( 'NONE', #5683, 1000.000000000000000 ) ;
#4139=ORIENTED_EDGE ( 'NONE', *, *, #4125, .T. ) ;
#4141=SHAPE_REPRESENTATION_RELATIONSHIP ( 'NONE' , 'NONE' ,  #3150, #2149 ) ;
#4143=CYLINDRICAL_SURFACE ( 'NONE', #656, 6.500000000000001776 ) ;
#4145=DIRECTION ( 'NONE',  ( 0.9999836672264332815, -0.005715354789859936752, 0.000000000000000000 ) ) ;
#4146=DIRECTION ( 'NONE',  ( 0.9999836672264333925, -0.005715354789860572528, 0.000000000000000000 ) ) ;
#4153=DIRECTION ( 'NONE',  ( -0.9979653668924883814, 0.06375834441969779887, 5.805357692931203648E-17 ) ) ;
#4159=CARTESIAN_POINT ( 'NONE',  ( -17.04733905648494030, -8.234069079964159599, -8.331366185709195643E-15 ) ) ;
#4163=DIRECTION ( 'NONE',  ( 0.9999836672264332815, -0.005715354789859936752, 0.000000000000000000 ) ) ;
#4166=VERTEX_POINT ( 'NONE', #4835 ) ;
#4168=DIRECTION ( 'NONE',  ( -5.715354789860003484E-18, -9.999836672264337477E-16, 1.000000000000000000 ) ) ;
#4178=CARTESIAN_POINT ( 'NONE',  ( -17.04733905648494030, -8.234069079964157822, -3.000000000000009326 ) ) ;
#4180=LINE ( 'NONE', #1905, #4814 ) ;
#4189=CARTESIAN_POINT ( 'NONE',  ( 35.76131148831677109, 4.835142255982176174, -2.999999999999995559 ) ) ;
#4192=CYLINDRICAL_SURFACE ( 'NONE', #987, 140.0000000000000284 ) ;
#4193=CARTESIAN_POINT ( 'NONE',  ( 0.000000000000000000, 0.000000000000000000, 0.000000000000000000 ) ) ;
#4194=ORIENTED_EDGE ( 'NONE', *, *, #4580, .T. ) ;
#4196=ORIENTED_EDGE ( 'NONE', *, *, #761, .T. ) ;
#4197=EDGE_CURVE ( 'NONE', #4894, #2728, #3596, .T. ) ;
#4198=PLANE ( 'NONE',  #2330 ) ;
#4207=AXIS2_PLACEMENT_3D ( 'NONE', #2257, #3645, #4712 ) ;
#4209=( LENGTH_UNIT ( ) NAMED_UNIT ( * ) SI_UNIT ( .MILLI., .METRE. ) );
#4212=VECTOR ( 'NONE', #2135, 1000.000000000000000 ) ;
#4216=VECTOR ( 'NONE', #6813, 1000.000000000000114 ) ;
#4226=CARTESIAN_POINT ( 'NONE',  ( 35.41737116972092281, 6.499986109694644298, -1.499999999999993783 ) ) ;
#4229=ORIENTED_EDGE ( 'NONE', *, *, #4580, .F. ) ;
#4231=VECTOR ( 'NONE', #1491, 1000.000000000000000 ) ;
#4257=DIRECTION ( 'NONE',  ( 0.9999836672264331705, -0.005715354789860001804, 0.000000000000000000 ) ) ;
#4260=( GEOMETRIC_REPRESENTATION_CONTEXT ( 3 ) GLOBAL_UNCERTAINTY_ASSIGNED_CONTEXT ( ( #797 ) ) GLOBAL_UNIT_ASSIGNED_CONTEXT ( ( #6381, #3076, #6349 ) ) REPRESENTATION_CONTEXT ( 'NONE', 'WORKASPACE' ) );
#4263=EDGE_CURVE ( 'NONE', #7025, #878, #2751, .T. ) ;
#4264=EDGE_CURVE ( 'NONE', #4598, #3100, #1557, .T. ) ;
#4268=CARTESIAN_POINT ( 'NONE',  ( 104.0973215944787711, -119.5240462704291389, -3.000000000000119904 ) ) ;
#4278=VERTEX_POINT ( 'NONE', #2783 ) ;
#4283=VERTEX_POINT ( 'NONE', #5102 ) ;
#4290=CARTESIAN_POINT ( 'NONE',  ( -12.10129460565897475, -12.45149060151658382, -1.252045042622798671E-14 ) ) ;
#4292=EDGE_LOOP ( 'NONE', ( #3886, #415, #6647, #4491 ) ) ;
#4298=CARTESIAN_POINT ( 'NONE',  ( -13.19674249314596892, -2.997380612392111843, -3.000000000000003997 ) ) ;
#4303=EDGE_CURVE ( 'NONE', #4319, #3409, #2679, .T. ) ;
#4305=CARTESIAN_POINT ( 'NONE',  ( -14.38395162568175145, 6.352317343304507702, 6.270004205522762891E-15 ) ) ;
#4319=VERTEX_POINT ( 'NONE', #4986 ) ;
#4326=VECTOR ( 'NONE', #5014, 1000.000000000000000 ) ;
#4327=EDGE_LOOP ( 'NONE', ( #587, #1562, #2588, #5129 ) ) ;
#4335=AXIS2_PLACEMENT_3D ( 'NONE', #2827, #5709, #1747 ) ;
#4345=DIRECTION ( 'NONE',  ( 0.9999836672264332815, -0.005715354789860001804, 0.000000000000000000 ) ) ;
#4349=DIRECTION ( 'NONE',  ( 5.715354789860003484E-18, 9.999836672264337477E-16, -1.000000000000000000 ) ) ;
#4360=CIRCLE ( 'NONE', #4735, 1.100000000000000755 ) ;
#4363=CARTESIAN_POINT ( 'NONE',  ( -12.20412794045469518, -35.68083184586667045, -3.000000000000036415 ) ) ;
#4365=LINE ( 'NONE', #897, #6651 ) ;
#4367=VECTOR ( 'NONE', #4090, 1000.000000000000114 ) ;
#4368=VECTOR ( 'NONE', #3458, 999.9999999999998863 ) ;
#4369=VECTOR ( 'NONE', #2333, 1000.000000000000114 ) ;
#4372=AXIS2_PLACEMENT_3D ( 'NONE', #4773, #3629, #3700 ) ;
#4374=AXIS2_PLACEMENT_3D ( 'NONE', #5004, #4435, #2123 ) ;
#4375=AXIS2_PLACEMENT_3D ( 'NONE', #2439, #2916, #4677 ) ;
#4383=CARTESIAN_POINT ( 'NONE',  ( -33.25476684253234794, 13.81160679460617757, -1.499999999999986899 ) ) ;
#4393=FACE_OUTER_BOUND ( 'NONE', #2470, .T. ) ;
#4398=ORIENTED_EDGE ( 'NONE', *, *, #1031, .T. ) ;
#4399=ORIENTED_EDGE ( 'NONE', *, *, #1437, .F. ) ;
#4405=DIRECTION ( 'NONE',  ( -5.715354789860003484E-18, -9.999836672264337477E-16, 1.000000000000000000 ) ) ;
#4409=DIRECTION ( 'NONE',  ( -0.9793199139485103677, -0.2023178344681514362, -2.079116908177635377E-16 ) ) ;
#4415=EDGE_LOOP ( 'NONE', ( #1927, #1679, #5568, #6465 ) ) ;
#4417=CYLINDRICAL_SURFACE ( 'NONE', #2779, 1.100000000000000755 ) ;
#4423=ORIENTED_EDGE ( 'NONE', *, *, #1437, .T. ) ;
#4431=ADVANCED_FACE ( 'NONE', ( #5216 ), #88, .F. ) ;
#4435=DIRECTION ( 'NONE',  ( -0.9147661038495488173, 0.4039838799357178822, 0.000000000000000000 ) ) ;
#4437=DIRECTION ( 'NONE',  ( -5.715354789860003484E-18, -9.999836672264337477E-16, 1.000000000000000000 ) ) ;
#4441=EDGE_CURVE ( 'NONE', #5643, #5379, #4656, .T. ) ;
#4442=ORIENTED_EDGE ( 'NONE', *, *, #1963, .T. ) ;
#4443=DIRECTION ( 'NONE',  ( -0.4039838799357176602, -0.9147661038495489283, -9.170600743851254660E-16 ) ) ;
#4447=DIRECTION ( 'NONE',  ( 0.9858503002877112564, -0.1676281164441980331, -1.619908943762944784E-16 ) ) ;
#4448=DIRECTION ( 'NONE',  ( 0.9999836672264332815, -0.005715354789859183882, 0.000000000000000000 ) ) ;
#4449=EDGE_CURVE ( 'NONE', #6990, #6323, #3999, .T. ) ;
#4453=CARTESIAN_POINT ( 'NONE',  ( -12.75609440306747189, -34.09959597428994726, -3.000000000000035083 ) ) ;
#4465=LINE ( 'NONE', #2239, #2066 ) ;
#4471=ORIENTED_EDGE ( 'NONE', *, *, #5502, .F. ) ;
#4480=CIRCLE ( 'NONE', #3529, 3.750000000000000444 ) ;
#4483=PLANE ( 'NONE',  #44 ) ;
#4485=ADVANCED_FACE ( 'NONE', ( #2379 ), #5255, .T. ) ;
#4487=CIRCLE ( 'NONE', #1595, 1.100000000000000755 ) ;
#4491=ORIENTED_EDGE ( 'NONE', *, *, #1269, .F. ) ;
#4493=CIRCLE ( 'NONE', #2914, 140.0000000000000284 ) ;
#4497=EDGE_CURVE ( 'NONE', #2788, #6066, #6855, .T. ) ;
#4501=CIRCLE ( 'NONE', #1931, 0.7500000000000000000 ) ;
#4504=AXIS2_PLACEMENT_3D ( 'NONE', #5781, #4614, #155 ) ;
#4505=AXIS2_PLACEMENT_3D ( 'NONE', #1772, #3460, #4145 ) ;
#4507=CARTESIAN_POINT ( 'NONE',  ( -35.54168210215660650, 14.82156649444490348, -0.7500000000019999558 ) ) ;
#4518=EDGE_LOOP ( 'NONE', ( #2002, #3914 ) ) ;
#4520=CARTESIAN_POINT ( 'NONE',  ( -44.78727511552453677, -94.39397278840091587, -3.000000000000095479 ) ) ;
#4523=CARTESIAN_POINT ( 'NONE',  ( 1.714606436958001585E-17, 2.999951001679301835E-15, -3.000000000000000888 ) ) ;
#4530=CARTESIAN_POINT ( 'NONE',  ( -28.22553731214382111, -35.79092421365019305, -3.000000000000036859 ) ) ;
#4532=EDGE_CURVE ( 'NONE', #5341, #6990, #684, .T. ) ;
#4537=CARTESIAN_POINT ( 'NONE',  ( -16.51707533432788111, -40.85914143033993895, -4.095287503286137508E-14 ) ) ;
#4539=EDGE_CURVE ( 'NONE', #937, #1893, #3545, .T. ) ;
#4555=FACE_OUTER_BOUND ( 'NONE', #3075, .T. ) ;
#4559=EDGE_CURVE ( 'NONE', #1044, #4778, #496, .T. ) ;
#4561=DIRECTION ( 'NONE',  ( -5.715354789860003484E-18, -9.999836672264337477E-16, 1.000000000000000000 ) ) ;
#4565=FACE_OUTER_BOUND ( 'NONE', #952, .T. ) ;
#4571=DIRECTION ( 'NONE',  ( 0.9999836672264332815, -0.005715354789859975783, 0.000000000000000000 ) ) ;
#4574=ORIENTED_EDGE ( 'NONE', *, *, #3271, .F. ) ;
#4580=EDGE_CURVE ( 'NONE', #1914, #4962, #975, .T. ) ;
#4589=CARTESIAN_POINT ( 'NONE',  ( -32.93157973858376408, 14.54341967768581512, 1.435496648130876646E-14 ) ) ;
#4591=DIRECTION ( 'NONE',  ( 0.9999836672264332815, -0.005715354789859936752, 0.000000000000000000 ) ) ;
#4594=CARTESIAN_POINT ( 'NONE',  ( -44.78727511552453677, -94.39397278840091587, -3.001000000000095813 ) ) ;
#4595=AXIS2_PLACEMENT_3D ( 'NONE', #4537, #2785, #5559 ) ;
#4598=VERTEX_POINT ( 'NONE', #4979 ) ;
#4599=ORIENTED_EDGE ( 'NONE', *, *, #2695, .T. ) ;
#4603=FACE_OUTER_BOUND ( 'NONE', #304, .T. ) ;
#4611=DIRECTION ( 'NONE',  ( 0.9999836672264332815, -0.005715354789860000936, 0.000000000000000000 ) ) ;
#4612=DIRECTION ( 'NONE',  ( -5.715354789860003484E-18, -9.999836672264337477E-16, 1.000000000000000000 ) ) ;
#4614=DIRECTION ( 'NONE',  ( 5.715354789860003484E-18, 9.999836672264337477E-16, -1.000000000000000000 ) ) ;
#4616=AXIS2_PLACEMENT_3D ( 'NONE', #3699, #730, #100 ) ;
#4620=CYLINDRICAL_SURFACE ( 'NONE', #2315, 1.100000000000000755 ) ;
#4622=VECTOR ( 'NONE', #7050, 1000.000000000000114 ) ;
#4636=DIRECTION ( 'NONE',  ( -5.715354789860003484E-18, -9.999836672264337477E-16, 1.000000000000000000 ) ) ;
#4643=EDGE_CURVE ( 'NONE', #4166, #5010, #5423, .T. ) ;
#4644=EDGE_CURVE ( 'NONE', #3100, #6678, #6086, .T. ) ;
#4646=CARTESIAN_POINT ( 'NONE',  ( -12.20412794045469518, -35.68083184586667045, -3.575000000000001175E-14 ) ) ;
#4647=DIRECTION ( 'NONE',  ( 0.9999836672264332815, -0.005715354789860036498, 0.000000000000000000 ) ) ;
#4655=CARTESIAN_POINT ( 'NONE',  ( 1.714606436958001585E-17, 2.999951001679301835E-15, -3.000000000000000888 ) ) ;
#4656=LINE ( 'NONE', #53, #2882 ) ;
#4658=ORIENTED_EDGE ( 'NONE', *, *, #2996, .T. ) ;
#4659=DIRECTION ( 'NONE',  ( -5.715354789860003484E-18, -9.999836672264337477E-16, 1.000000000000000000 ) ) ;
#4660=FILL_AREA_STYLE ('',( #2557 ) ) ;
#4664=DIRECTION ( 'NONE',  ( 0.9999836672264332815, -0.005715354789859183882, 0.000000000000000000 ) ) ;
#4667=ORIENTED_EDGE ( 'NONE', *, *, #7423, .T. ) ;
#4677=DIRECTION ( 'NONE',  ( 0.9999836672264332815, -0.005715354789859956701, 0.000000000000000000 ) ) ;
#4680=EDGE_CURVE ( 'NONE', #6339, #461, #908, .T. ) ;
#4687=EDGE_CURVE ( 'NONE', #3571, #5033, #3718, .T. ) ;
#4689=ORIENTED_EDGE ( 'NONE', *, *, #4072, .F. ) ;
#4696=ORIENTED_EDGE ( 'NONE', *, *, #2521, .T. ) ;
#4698=ORIENTED_EDGE ( 'NONE', *, *, #4303, .T. ) ;
#4700=LINE ( 'NONE', #6432, #5585 ) ;
#4705=EDGE_LOOP ( 'NONE', ( #2944, #2343, #3215, #7024 ) ) ;
#4706=VERTEX_POINT ( 'NONE', #4942 ) ;
#4711=DIRECTION ( 'NONE',  ( 5.715354789860003484E-18, 9.999836672264337477E-16, -1.000000000000000000 ) ) ;
#4712=DIRECTION ( 'NONE',  ( 0.9999836672264331705, -0.005715354789860001804, 0.000000000000000000 ) ) ;
#4716=CARTESIAN_POINT ( 'NONE',  ( 12.26605808802378661, -5.710507655519337256, -5.640309513244763609E-15 ) ) ;
#4719=DIRECTION ( 'NONE',  ( 0.9999836672264331705, -0.005715354789859876036, 0.000000000000000000 ) ) ;
#4721=CIRCLE ( 'NONE', #2176, 2.250000000000031974 ) ;
#4723=AXIS2_PLACEMENT_3D ( 'NONE', #4268, #970, #5931 ) ;
#4728=VECTOR ( 'NONE', #1247, 1000.000000000000000 ) ;
#4733=ORIENTED_EDGE ( 'NONE', *, *, #3293, .F. ) ;
#4735=AXIS2_PLACEMENT_3D ( 'NONE', #411, #5005, #4591 ) ;
#4738=ORIENTED_EDGE ( 'NONE', *, *, #4559, .T. ) ;
#4744=AXIS2_PLACEMENT_3D ( 'NONE', #4001, #3435, #5217 ) ;
#4745=EDGE_LOOP ( 'NONE', ( #1450, #2358, #5775 ) ) ;
#4763=DIRECTION ( 'NONE',  ( 0.9999836672264332815, -0.005715354789859975783, 0.000000000000000000 ) ) ;
#4764=EDGE_CURVE ( 'NONE', #6339, #5766, #6263, .T. ) ;
#4773=CARTESIAN_POINT ( 'NONE',  ( -16.51707533432788111, -40.85914143033993895, -4.095287503286137508E-14 ) ) ;
#4777=ADVANCED_FACE ( 'NONE', ( #5136 ), #3606, .F. ) ;
#4778=VERTEX_POINT ( 'NONE', #4069 ) ;
#4781=FACE_OUTER_BOUND ( 'NONE', #4745, .T. ) ;
#4784=CARTESIAN_POINT ( 'NONE',  ( -32.93157973858376408, 14.54341967768581867, -2.999999999999986677 ) ) ;
#4790=CARTESIAN_POINT ( 'NONE',  ( -8.617355793880991044, 7.615193964809151339, 7.565818341857973962E-15 ) ) ;
#4794=LINE ( 'NONE', #3579, #1114 ) ;
#4795=EDGE_CURVE ( 'NONE', #6066, #364, #2853, .T. ) ;
#4796=CARTESIAN_POINT ( 'NONE',  ( -13.60410507457170226, -35.67283034916086848, -3.575000000000001175E-14 ) ) ;
#4800=DIRECTION ( 'NONE',  ( -5.715354789860003484E-18, -9.999836672264337477E-16, 1.000000000000000000 ) ) ;
#4802=ORIENTED_EDGE ( 'NONE', *, *, #5590, .T. ) ;
#4805=EDGE_CURVE ( 'NONE', #6323, #5266, #2293, .T. ) ;
#4808=CARTESIAN_POINT ( 'NONE',  ( -41.31559769795914150, -94.79889909491285493, -3.001000000000096257 ) ) ;
#4810=ORIENTED_EDGE ( 'NONE', *, *, #6555, .F. ) ;
#4814=VECTOR ( 'NONE', #6996, 1000.000000000000114 ) ;
#4817=LINE ( 'NONE', #7036, #5212 ) ;
#4819=AXIS2_PLACEMENT_3D ( 'NONE', #2740, #6226, #1060 ) ;
#4824=DIRECTION ( 'NONE',  ( -5.715354789860003484E-18, -9.999836672264337477E-16, 1.000000000000000000 ) ) ;
#4826=LINE ( 'NONE', #7362, #1242 ) ;
#4835=CARTESIAN_POINT ( 'NONE',  ( -3.749938752099124972, 0.02143258046197846906, -3.000000000000000888 ) ) ;
#4837=CARTESIAN_POINT ( 'NONE',  ( -28.26870112771624832, 11.60963389179610594, -1.499999999999988898 ) ) ;
#4838=CIRCLE ( 'NONE', #1952, 5.000000000000001776 ) ;
#4842=VERTEX_POINT ( 'NONE', #6852 ) ;
#4849=EDGE_CURVE ( 'NONE', #3970, #74, #3495, .T. ) ;
#4854=CARTESIAN_POINT ( 'NONE',  ( 30.52077159997899969, 5.488396937354000471, -1.500000000001999956 ) ) ;
#4863=ORIENTED_EDGE ( 'NONE', *, *, #4449, .F. ) ;
#4866=CYLINDRICAL_SURFACE ( 'NONE', #394, 3.750000000000000444 ) ;
#4870=CARTESIAN_POINT ( 'NONE',  ( 94.42889356597736139, -103.2882618349535591, -3.000000000000103917 ) ) ;
#4879=PRODUCT_DEFINITION_CONTEXT ( 'detailed design', #6777, 'design' ) ;
#4883=VERTEX_POINT ( 'NONE', #3291 ) ;
#4885=ORIENTED_EDGE ( 'NONE', *, *, #2504, .F. ) ;
#4886=PLANE ( 'NONE',  #2547 ) ;
#4889=CARTESIAN_POINT ( 'NONE',  ( -40.65229780501017842, -93.90085982332455217, -3.001000000000095369 ) ) ;
#4893=ORIENTED_EDGE ( 'NONE', *, *, #910, .F. ) ;
#4894=VERTEX_POINT ( 'NONE', #2755 ) ;
#4898=DIRECTION ( 'NONE',  ( -0.9999836672264333925, 0.005715354789860572528, 0.000000000000000000 ) ) ;
#4904=EDGE_CURVE ( 'NONE', #1452, #1493, #2154, .T. ) ;
#4925=CARTESIAN_POINT ( 'NONE',  ( -13.60410507457170226, -35.67283034916086848, -3.000000000000036415 ) ) ;
#4928=ORIENTED_EDGE ( 'NONE', *, *, #3987, .F. ) ;
#4935=ORIENTED_EDGE ( 'NONE', *, *, #6022, .T. ) ;
#4942=CARTESIAN_POINT ( 'NONE',  ( -45.21893524706405287, -93.36435596057614816, -9.362127331984775681E-14 ) ) ;
#4943=AXIS2_PLACEMENT_3D ( 'NONE', #2910, #5295, #3016 ) ;
#4951=ORIENTED_EDGE ( 'NONE', *, *, #2234, .F. ) ;
#4954=ORIENTED_EDGE ( 'NONE', *, *, #429, .T. ) ;
#4955=LINE ( 'NONE', #322, #5468 ) ;
#4961=ORIENTED_EDGE ( 'NONE', *, *, #4643, .T. ) ;
#4962=VERTEX_POINT ( 'NONE', #6209 ) ;
#4965=DIRECTION ( 'NONE',  ( -5.715354789860003484E-18, -9.999836672264337477E-16, 1.000000000000000000 ) ) ;
#4966=COLOUR_RGB ( '', 0.40784314, 0.44705882, 0.49803922) ;
#4967=FACE_OUTER_BOUND ( 'NONE', #945, .T. ) ;
#4972=ADVANCED_FACE ( 'NONE', ( #2798 ), #7396, .T. ) ;
#4977=AXIS2_PLACEMENT_3D ( 'NONE', #849, #6503, #1349 ) ;
#4979=CARTESIAN_POINT ( 'NONE',  ( 15.39900769062488806, 3.181283097128406290, -2.999999999999997335 ) ) ;
#4982=AXIS2_PLACEMENT_3D ( 'NONE', #7271, #2110, #3355 ) ;
#4986=CARTESIAN_POINT ( 'NONE',  ( -14.38395162568175145, 6.352317343304510366, -2.999999999999994671 ) ) ;
#4991=ORIENTED_EDGE ( 'NONE', *, *, #3838, .F. ) ;
#4993=CARTESIAN_POINT ( 'NONE',  ( -10.41850315652351533, -32.21925899276746463, -3.000000000000032863 ) ) ;
#4995=EDGE_CURVE ( 'NONE', #3340, #5544, #6455, .T. ) ;
#5000=ORIENTED_EDGE ( 'NONE', *, *, #3799, .F. ) ;
#5003=ORIENTED_EDGE ( 'NONE', *, *, #4539, .F. ) ;
#5004=CARTESIAN_POINT ( 'NONE',  ( -28.68093632328499965, 11.79168739492699913, -1.500000000001999956 ) ) ;
#5005=DIRECTION ( 'NONE',  ( -5.715354789860003484E-18, -9.999836672264337477E-16, 1.000000000000000000 ) ) ;
#5009=ORIENTED_EDGE ( 'NONE', *, *, #5283, .F. ) ;
#5010=VERTEX_POINT ( 'NONE', #2463 ) ;
#5014=DIRECTION ( 'NONE',  ( -5.715354789860003484E-18, -9.999836672264337477E-16, 1.000000000000000000 ) ) ;
#5019=DIRECTION ( 'NONE',  ( 1.387778780781445676E-14, 2.775557561562891351E-14, 1.000000000000000000 ) ) ;
#5027=CARTESIAN_POINT ( 'NONE',  ( 35.76131148831677109, 4.835142255982173509, 5.039451867604972471E-15 ) ) ;
#5033=VERTEX_POINT ( 'NONE', #620 ) ;
#5038=DIRECTION ( 'NONE',  ( 0.4039838799357177157, 0.9147661038495489283, 9.170600743851256632E-16 ) ) ;
#5039=PLANE ( 'NONE',  #7132 ) ;
#5042=ORIENTED_EDGE ( 'NONE', *, *, #1269, .T. ) ;
#5053=ORIENTED_EDGE ( 'NONE', *, *, #4680, .F. ) ;
#5054=EDGE_CURVE ( 'NONE', #3671, #3409, #248, .T. ) ;
#5055=AXIS2_PLACEMENT_3D ( 'NONE', #3602, #5916, #4146 ) ;
#5073=ORIENTED_EDGE ( 'NONE', *, *, #5147, .T. ) ;
#5076=DIRECTION ( 'NONE',  ( 5.715354789860003484E-18, 9.999836672264337477E-16, -1.000000000000000000 ) ) ;
#5078=CARTESIAN_POINT ( 'NONE',  ( -40.65229780501022816, -93.90085982332443848, -3.000000000000095035 ) ) ;
#5081=VERTEX_POINT ( 'NONE', #7019 ) ;
#5084=CARTESIAN_POINT ( 'NONE',  ( -19.94212619460468261, -40.63668738334721553, -4.075000000000002200E-14 ) ) ;
#5088=CIRCLE ( 'NONE', #1121, 2.500000000000000000 ) ;
#5090=EDGE_CURVE ( 'NONE', #5010, #1273, #6980, .T. ) ;
#5099=DIRECTION ( 'NONE',  ( 0.9793199139485100346, 0.2023178344681531293, 1.787644449902631965E-16 ) ) ;
#5102=CARTESIAN_POINT ( 'NONE',  ( -41.31559769795914150, -94.79889909491285493, -9.503348406515855143E-14 ) ) ;
#5105=AXIS2_PLACEMENT_3D ( 'NONE', #3468, #6375, #5320 ) ;
#5106=AXIS2_PLACEMENT_3D ( 'NONE', #6092, #7065, #3804 ) ;
#5118=ORIENTED_EDGE ( 'NONE', *, *, #2996, .F. ) ;
#5129=ORIENTED_EDGE ( 'NONE', *, *, #5090, .F. ) ;
#5136=FACE_OUTER_BOUND ( 'NONE', #3295, .T. ) ;
#5138=EDGE_CURVE ( 'NONE', #6678, #3671, #3120, .T. ) ;
#5139=EDGE_CURVE ( 'NONE', #878, #3729, #4098, .T. ) ;
#5144=CARTESIAN_POINT ( 'NONE',  ( -28.70619392989860330, -36.67182071578998404, -3.001000000000038082 ) ) ;
#5145=ORIENTED_EDGE ( 'NONE', *, *, #1774, .T. ) ;
#5147=EDGE_CURVE ( 'NONE', #2280, #74, #1814, .T. ) ;
#5160=ORIENTED_EDGE ( 'NONE', *, *, #1040, .T. ) ;
#5170=DIRECTION ( 'NONE',  ( -0.2023178344681547114, 0.9793199139485095905, 8.673617379884032514E-16 ) ) ;
#5171=ORIENTED_EDGE ( 'NONE', *, *, #5378, .T. ) ;
#5176=ADVANCED_FACE ( 'NONE', ( #3585, #5900, #725 ), #5332, .F. ) ;
#5180=DIRECTION ( 'NONE',  ( 0.9999836672264332815, -0.005715354789859936752, 0.000000000000000000 ) ) ;
#5181=SURFACE_STYLE_FILL_AREA ( #4660 ) ;
#5190=EDGE_LOOP ( 'NONE', ( #4667, #1657, #21, #4951 ) ) ;
#5193=CARTESIAN_POINT ( 'NONE',  ( -44.78727511552453677, -94.39397278840091587, -9.464840624037363205E-14 ) ) ;
#5199=ORIENTED_EDGE ( 'NONE', *, *, #7423, .F. ) ;
#5201=CARTESIAN_POINT ( 'NONE',  ( -20.89962323070193406, -41.21687045383659154, -3.000000000000042188 ) ) ;
#5211=VECTOR ( 'NONE', #5595, 1000.000000000000000 ) ;
#5212=VECTOR ( 'NONE', #3566, 1000.000000000000000 ) ;
#5216=FACE_OUTER_BOUND ( 'NONE', #4415, .T. ) ;
#5217=DIRECTION ( 'NONE',  ( -0.2023178344681547114, 0.9793199139485095905, 8.673617379884032514E-16 ) ) ;
#5219=VECTOR ( 'NONE', #3332, 1000.000000000000000 ) ;
#5220=VERTEX_POINT ( 'NONE', #4837 ) ;
#5223=DIRECTION ( 'NONE',  ( 0.9999836672264331705, -0.005715354789860001804, 0.000000000000000000 ) ) ;
#5227=LINE ( 'NONE', #5277, #2787 ) ;
#5233=ORIENTED_EDGE ( 'NONE', *, *, #6831, .F. ) ;
#5234=EDGE_LOOP ( 'NONE', ( #726, #5726 ) ) ;
#5237=ORIENTED_EDGE ( 'NONE', *, *, #5138, .T. ) ;
#5247=CARTESIAN_POINT ( 'NONE',  ( -20.89962323070193406, -41.21687045383659154, -3.000000000000042188 ) ) ;
#5248=CARTESIAN_POINT ( 'NONE',  ( -15.80406914246985650, -35.66025656862317561, -3.000000000000036415 ) ) ;
#5255=CYLINDRICAL_SURFACE ( 'NONE', #4335, 0.7499999999999994449 ) ;
#5261=CARTESIAN_POINT ( 'NONE',  ( -28.70619392989860330, -36.67182071578998404, -3.000000000000037748 ) ) ;
#5265=DIRECTION ( 'NONE',  ( 0.9999836672264331705, -0.005715354789860049509, 0.000000000000000000 ) ) ;
#5266=VERTEX_POINT ( 'NONE', #240 ) ;
#5277=CARTESIAN_POINT ( 'NONE',  ( 30.36903322412724293, 6.222886872815265313, -1.499999999999994227 ) ) ;
#5283=EDGE_CURVE ( 'NONE', #5220, #7266, #7085, .T. ) ;
#5288=CARTESIAN_POINT ( 'NONE',  ( 94.42889356597736139, -103.2882618349535591, -3.000000000000103917 ) ) ;
#5290=ADVANCED_FACE ( 'NONE', ( #3060 ), #5980, .F. ) ;
#5291=EDGE_LOOP ( 'NONE', ( #487, #3685, #3853, #449 ) ) ;
#5295=DIRECTION ( 'NONE',  ( 5.715354789860003484E-18, 9.999836672264337477E-16, -1.000000000000000000 ) ) ;
#5300=CARTESIAN_POINT ( 'NONE',  ( -10.54744521951312208, -8.271218886098244738, -3.000000000000009326 ) ) ;
#5304=EDGE_LOOP ( 'NONE', ( #7092, #6807 ) ) ;
#5305=ORIENTED_EDGE ( 'NONE', *, *, #837, .T. ) ;
#5320=DIRECTION ( 'NONE',  ( -0.9999836672264332815, 0.005715354789860036498, 0.000000000000000000 ) ) ;
#5321=ORIENTED_EDGE ( 'NONE', *, *, #4532, .F. ) ;
#5332=PLANE ( 'NONE',  #6984 ) ;
#5333=ORIENTED_EDGE ( 'NONE', *, *, #4680, .T. ) ;
#5341=VERTEX_POINT ( 'NONE', #2077 ) ;
#5342=CONICAL_SURFACE ( 'NONE', #759, 0.7499999999999863443, 1.029744258676653645 ) ;
#5343=DIRECTION ( 'NONE',  ( -5.715354789860003484E-18, -9.999836672264337477E-16, 1.000000000000000000 ) ) ;
#5348=CONICAL_SURFACE ( 'NONE', #4744, 0.7500000000000002220, 1.029744258676651425 ) ;
#5365=ORIENTED_EDGE ( 'NONE', *, *, #5502, .T. ) ;
#5378=EDGE_CURVE ( 'NONE', #3100, #6173, #2414, .T. ) ;
#5379=VERTEX_POINT ( 'NONE', #2230 ) ;
#5384=ORIENTED_EDGE ( 'NONE', *, *, #836, .T. ) ;
#5385=ORIENTED_EDGE ( 'NONE', *, *, #4805, .F. ) ;
#5397=DIRECTION ( 'NONE',  ( -5.715354789860003484E-18, -9.999836672264337477E-16, 1.000000000000000000 ) ) ;
#5399=EDGE_CURVE ( 'NONE', #1922, #2186, #3611, .T. ) ;
#5400=UNCERTAINTY_MEASURE_WITH_UNIT (LENGTH_MEASURE( 1.000000000000000082E-05 ), #4209, 'distance_accuracy_value', 'NONE');
#5414=ORIENTED_EDGE ( 'NONE', *, *, #5477, .T. ) ;
#5423=CIRCLE ( 'NONE', #4819, 3.750000000000000444 ) ;
#5424=DIRECTION ( 'NONE',  ( -0.9147661038495489283, 0.4039838799357176602, 3.987490689252441100E-16 ) ) ;
#5428=CARTESIAN_POINT ( 'NONE',  ( 7.283874945971848369, -8.906884184084093548, -3.000000000000009770 ) ) ;
#5430=EDGE_CURVE ( 'NONE', #1273, #7056, #2926, .T. ) ;
#5467=PLANE ( 'NONE',  #5851 ) ;
#5468=VECTOR ( 'NONE', #1600, 1000.000000000000000 ) ;
#5477=EDGE_CURVE ( 'NONE', #4883, #3069, #2265, .T. ) ;
#5487=EDGE_CURVE ( 'NONE', #3871, #1452, #6785, .T. ) ;
#5502=EDGE_CURVE ( 'NONE', #7163, #7292, #3921, .T. ) ;
#5511=CARTESIAN_POINT ( 'NONE',  ( 10.02759472486470926, 5.630039434485816230, 5.687258741868093102E-15 ) ) ;
#5513=EDGE_LOOP ( 'NONE', ( #1921, #4885 ) ) ;
#5516=DIRECTION ( 'NONE',  ( 0.9999836672264331705, -0.005715354789860049509, 0.000000000000000000 ) ) ;
#5519=CARTESIAN_POINT ( 'NONE',  ( 104.0973215944787711, -119.5240462704291389, -1.189271409856590718E-13 ) ) ;
#5521=DIRECTION ( 'NONE',  ( -0.9147661038495482622, 0.4039838799357193255, 3.987490689252457863E-16 ) ) ;
#5523=DIRECTION ( 'NONE',  ( -5.715354789860003484E-18, -9.999836672264337477E-16, 1.000000000000000000 ) ) ;
#5526=CARTESIAN_POINT ( 'NONE',  ( 14.38741851828413942, 8.077882666870964457, -2.999999999999992895 ) ) ;
#5541=DIRECTION ( 'NONE',  ( 5.715354789860003484E-18, 9.999836672264337477E-16, -1.000000000000000000 ) ) ;
#5543=AXIS2_PLACEMENT_3D ( 'NONE', #4226, #6524, #2029 ) ;
#5544=VERTEX_POINT ( 'NONE', #55 ) ;
#5546=DIRECTION ( 'NONE',  ( -0.1248576012279780517, 0.9921746718272922427, 1.096417580487671857E-15 ) ) ;
#5548=VECTOR ( 'NONE', #3267, 1000.000000000000000 ) ;
#5549=CARTESIAN_POINT ( 'NONE',  ( -32.93157973858376408, 14.54341967768581867, -2.999999999999986677 ) ) ;
#5553=ADVANCED_FACE ( 'NONE', ( #2299 ), #1186, .T. ) ;
#5554=EDGE_CURVE ( 'NONE', #5544, #6347, #5835, .T. ) ;
#5559=DIRECTION ( 'NONE',  ( 0.9999836672264333925, -0.005715354789860572528, 0.000000000000000000 ) ) ;
#5562=EDGE_CURVE ( 'NONE', #6173, #4319, #3532, .T. ) ;
#5568=ORIENTED_EDGE ( 'NONE', *, *, #3932, .T. ) ;
#5572=CONICAL_SURFACE ( 'NONE', #2908, 0.7499999999999863443, 1.029744258676653645 ) ;
#5578=VERTEX_POINT ( 'NONE', #6941 ) ;
#5585=VECTOR ( 'NONE', #1894, 1000.000000000000000 ) ;
#5588=FACE_OUTER_BOUND ( 'NONE', #3521, .T. ) ;
#5590=EDGE_CURVE ( 'NONE', #6756, #577, #286, .T. ) ;
#5591=EDGE_LOOP ( 'NONE', ( #4733, #7154 ) ) ;
#5593=VECTOR ( 'NONE', #6160, 1000.000000000000000 ) ;
#5594=STYLED_ITEM ( 'NONE', ( #6551 ), #7175 ) ;
#5595=DIRECTION ( 'NONE',  ( -0.8795363392562568494, 0.4758317222797389667, 4.707970883985391064E-16 ) ) ;
#5596=PLANE ( 'NONE',  #1003 ) ;
#5599=EDGE_CURVE ( 'NONE', #4842, #3938, #1256, .T. ) ;
#5611=ORIENTED_EDGE ( 'NONE', *, *, #4125, .F. ) ;
#5612=ORIENTED_EDGE ( 'NONE', *, *, #1023, .T. ) ;
#5618=DIRECTION ( 'NONE',  ( -5.715354789860003484E-18, -9.999836672264337477E-16, 1.000000000000000000 ) ) ;
#5623=CARTESIAN_POINT ( 'NONE',  ( 15.39900769062488806, 3.181283097128403625, 3.269241930315631824E-15 ) ) ;
#5633=DIRECTION ( 'NONE',  ( 0.9999836672264332815, -0.005715354789860000936, 0.000000000000000000 ) ) ;
#5634=ORIENTED_EDGE ( 'NONE', *, *, #1994, .F. ) ;
#5635=ORIENTED_EDGE ( 'NONE', *, *, #5430, .T. ) ;
#5638=DIRECTION ( 'NONE',  ( 0.9999836672264331705, -0.005715354789862803382, 0.000000000000000000 ) ) ;
#5643=VERTEX_POINT ( 'NONE', #2897 ) ;
#5646=ADVANCED_FACE ( 'NONE', ( #655 ), #5348, .F. ) ;
#5649=CARTESIAN_POINT ( 'NONE',  ( -10.54744521951312208, -8.271218886098244738, -3.000000000000009326 ) ) ;
#5660=ORIENTED_EDGE ( 'NONE', *, *, #979, .F. ) ;
#5661=VECTOR ( 'NONE', #2968, 999.9999999999998863 ) ;
#5662=EDGE_CURVE ( 'NONE', #5081, #7087, #3411, .T. ) ;
#5664=FACE_OUTER_BOUND ( 'NONE', #1892, .T. ) ;
#5669=ORIENTED_EDGE ( 'NONE', *, *, #5554, .F. ) ;
#5679=EDGE_CURVE ( 'NONE', #937, #6339, #5895, .T. ) ;
#5681=ORIENTED_EDGE ( 'NONE', *, *, #1775, .T. ) ;
#5683=DIRECTION ( 'NONE',  ( -0.3866393274467394559, 0.9222310071080526139, 9.200061635857666883E-16 ) ) ;
#5686=DIRECTION ( 'NONE',  ( 0.9999836672264331705, -0.005715354789862803382, 0.000000000000000000 ) ) ;
#5695=VECTOR ( 'NONE', #3, 1000.000000000000000 ) ;
#5698=DIRECTION ( 'NONE',  ( -5.715354789860003484E-18, -9.999836672264337477E-16, 1.000000000000000000 ) ) ;
#5704=VECTOR ( 'NONE', #6571, 999.9999999999998863 ) ;
#5705=AXIS2_PLACEMENT_3D ( 'NONE', #1722, #7401, #1122 ) ;
#5709=DIRECTION ( 'NONE',  ( -0.9793199139485100346, -0.2023178344681531293, -1.787644449902631965E-16 ) ) ;
#5722=DIRECTION ( 'NONE',  ( -0.4039838799357176602, -0.9147661038495489283, -9.170600743851254660E-16 ) ) ;
#5726=ORIENTED_EDGE ( 'NONE', *, *, #5872, .F. ) ;
#5727=PRODUCT_CONTEXT ( 'NONE', #6027, 'mechanical' ) ;
#5737=DIRECTION ( 'NONE',  ( 0.3309668111461608886, 0.9436423951475163552, 9.455185755993174392E-16 ) ) ;
#5738=ADVANCED_FACE ( 'NONE', ( #2571 ), #7118, .T. ) ;
#5758=ORIENTED_EDGE ( 'NONE', *, *, #1343, .F. ) ;
#5761=ADVANCED_FACE ( 'NONE', ( #3660 ), #795, .F. ) ;
#5766=VERTEX_POINT ( 'NONE', #236 ) ;
#5775=ORIENTED_EDGE ( 'NONE', *, *, #1362, .T. ) ;
#5777=DIRECTION ( 'NONE',  ( -0.4039838799357192700, -0.9147661038495482622, -8.673617379884158732E-16 ) ) ;
#5781=CARTESIAN_POINT ( 'NONE',  ( 104.0973215944787711, -119.5240462704291389, -3.000000000000119904 ) ) ;
#5793=ORIENTED_EDGE ( 'NONE', *, *, #3932, .F. ) ;
#5807=VERTEX_POINT ( 'NONE', #7412 ) ;
#5813=DIRECTION ( 'NONE',  ( 0.6778072752560848624, -0.7352396191786197965, -6.263809825053043546E-16 ) ) ;
#5831=VECTOR ( 'NONE', #6825, 1000.000000000000114 ) ;
#5835=CIRCLE ( 'NONE', #5105, 6.500000000000001776 ) ;
#5838=DIRECTION ( 'NONE',  ( 0.9999836672264332815, -0.005715354789860000936, 0.000000000000000000 ) ) ;
#5841=ORIENTED_EDGE ( 'NONE', *, *, #5679, .F. ) ;
#5844=CARTESIAN_POINT ( 'NONE',  ( -33.94153943842304955, 12.25650441806195801, -2.999999999999988898 ) ) ;
#5851=AXIS2_PLACEMENT_3D ( 'NONE', #7256, #297, #4405 ) ;
#5852=EDGE_LOOP ( 'NONE', ( #2231, #2313, #7441, #877 ) ) ;
#5872=EDGE_CURVE ( 'NONE', #6679, #5807, #176, .T. ) ;
#5881=PLANE ( 'NONE',  #3750 ) ;
#5882=CARTESIAN_POINT ( 'NONE',  ( -13.60410507457170226, -35.67283034916086848, -3.000000000000036415 ) ) ;
#5895=LINE ( 'NONE', #6521, #3044 ) ;
#5898=VECTOR ( 'NONE', #4447, 1000.000000000000114 ) ;
#5900=FACE_BOUND ( 'NONE', #853, .T. ) ;
#5904=ORIENTED_EDGE ( 'NONE', *, *, #5590, .F. ) ;
#5909=EDGE_CURVE ( 'NONE', #4166, #7056, #1058, .T. ) ;
#5913=CARTESIAN_POINT ( 'NONE',  ( 37.86567095459282228, 7.005780695865149177, -1.500000000001998623 ) ) ;
#5916=DIRECTION ( 'NONE',  ( -5.715354789860003484E-18, -9.999836672264337477E-16, 1.000000000000000000 ) ) ;
#5921=CLOSED_SHELL ( 'NONE', ( #3874, #5553, #6560, #1083, #4485, #4972, #7062, #7145, #4039, #5974, #6515, #5738, #6700, #319, #6329, #847, #2224, #3315, #6507, #2465, #1632, #3565, #5290, #6249, #1851, #6779, #5761, #4431, #4105, #7392, #5176, #2825, #2129, #6343, #6272, #1788, #3528, #2856, #3379, #4017, #7202, #3557 ) ) ;
#5925=EDGE_CURVE ( 'NONE', #6624, #4278, #1736, .T. ) ;
#5929=ORIENTED_EDGE ( 'NONE', *, *, #1650, .T. ) ;
#5931=DIRECTION ( 'NONE',  ( 0.9999836672264332815, -0.005715354789859956701, 0.000000000000000000 ) ) ;
#5939=CARTESIAN_POINT ( 'NONE',  ( -14.70408710852078116, -35.66654345889202204, -3.000000000000036415 ) ) ;
#5959=CARTESIAN_POINT ( 'NONE',  ( 0.000000000000000000, 0.000000000000000000, 0.000000000000000000 ) ) ;
#5962=AXIS2_PLACEMENT_3D ( 'NONE', #3085, #5397, #7157 ) ;
#5963=CARTESIAN_POINT ( 'NONE',  ( 35.41737116972092281, 6.499986109694644298, -1.499999999999993783 ) ) ;
#5974=ADVANCED_FACE ( 'NONE', ( #1287 ), #4143, .F. ) ;
#5979=CARTESIAN_POINT ( 'NONE',  ( -14.70408710852078116, -35.66654345889202204, -3.000000000000036415 ) ) ;
#5980=CYLINDRICAL_SURFACE ( 'NONE', #1923, 5.000000000000001776 ) ;
#5986=CARTESIAN_POINT ( 'NONE',  ( 35.53953323059130298, 5.908660390665234630, -1.055128867088183098 ) ) ;
#5990=ORIENTED_EDGE ( 'NONE', *, *, #5054, .F. ) ;
#5992=FACE_OUTER_BOUND ( 'NONE', #2500, .T. ) ;
#5997=VERTEX_POINT ( 'NONE', #5248 ) ;
#6005=DIRECTION ( 'NONE',  ( 0.5941197849118597940, 0.8043765792067080200, 8.077590468646243185E-16 ) ) ;
#6008=DIRECTION ( 'NONE',  ( -0.9147661038495488173, 0.4039838799357178822, 0.000000000000000000 ) ) ;
#6015=EDGE_LOOP ( 'NONE', ( #283, #1497 ) ) ;
#6019=FACE_BOUND ( 'NONE', #5513, .T. ) ;
#6022=EDGE_CURVE ( 'NONE', #1124, #3341, #2937, .T. ) ;
#6027=APPLICATION_CONTEXT ( 'automotive_design' ) ;
#6029=DIRECTION ( 'NONE',  ( -5.715354789860003484E-18, -9.999836672264337477E-16, 1.000000000000000000 ) ) ;
#6032=FACE_OUTER_BOUND ( 'NONE', #2316, .T. ) ;
#6054=ORIENTED_EDGE ( 'NONE', *, *, #4263, .T. ) ;
#6064=VERTEX_POINT ( 'NONE', #5882 ) ;
#6066=VERTEX_POINT ( 'NONE', #6994 ) ;
#6073=CIRCLE ( 'NONE', #164, 0.7500000000000000000 ) ;
#6075=LINE ( 'NONE', #7179, #529 ) ;
#6078=VECTOR ( 'NONE', #4437, 1000.000000000000000 ) ;
#6083=AXIS2_PLACEMENT_3D ( 'NONE', #7080, #3580, #3012 ) ;
#6084=ORIENTED_EDGE ( 'NONE', *, *, #439, .F. ) ;
#6086=LINE ( 'NONE', #6667, #3965 ) ;
#6088=ORIENTED_EDGE ( 'NONE', *, *, #1870, .T. ) ;
#6090=DIRECTION ( 'NONE',  ( 5.715354789860003484E-18, 9.999836672264337477E-16, -1.000000000000000000 ) ) ;
#6092=CARTESIAN_POINT ( 'NONE',  ( -17.04733905648494030, -8.234069079964157822, -3.000000000000009326 ) ) ;
#6109=CARTESIAN_POINT ( 'NONE',  ( 94.42889356597736139, -103.2882618349535591, -1.027468802220174526E-13 ) ) ;
#6110=CARTESIAN_POINT ( 'NONE',  ( -8.617355793880991044, 7.615193964809154004, -2.999999999999993339 ) ) ;
#6111=DIRECTION ( 'NONE',  ( -0.9147661038495495944, 0.4039838799357160504, 3.987490689252424829E-16 ) ) ;
#6123=LINE ( 'NONE', #868, #7129 ) ;
#6124=CARTESIAN_POINT ( 'NONE',  ( -14.38395162568175145, 6.352317343304510366, -2.999999999999994671 ) ) ;
#6127=DIRECTION ( 'NONE',  ( -5.715354789860003484E-18, -9.999836672264337477E-16, 1.000000000000000000 ) ) ;
#6136=ORIENTED_EDGE ( 'NONE', *, *, #1988, .F. ) ;
#6137=ORIENTED_EDGE ( 'NONE', *, *, #7022, .T. ) ;
#6144=ORIENTED_EDGE ( 'NONE', *, *, #2511, .T. ) ;
#6145=CIRCLE ( 'NONE', #3959, 0.7500000000000002220 ) ;
#6146=ORIENTED_EDGE ( 'NONE', *, *, #537, .F. ) ;
#6160=DIRECTION ( 'NONE',  ( -5.715354789860003484E-18, -9.999836672264337477E-16, 1.000000000000000000 ) ) ;
#6166=AXIS2_PLACEMENT_3D ( 'NONE', #2689, #6748, #2082 ) ;
#6173=VERTEX_POINT ( 'NONE', #6110 ) ;
#6175=AXIS2_PLACEMENT_3D ( 'NONE', #2288, #3344, #3380 ) ;
#6177=CARTESIAN_POINT ( 'NONE',  ( -19.94212619460463287, -40.63668738334721553, -3.000000000000041744 ) ) ;
#6183=DIRECTION ( 'NONE',  ( -0.8552446107963830313, -0.5182245224839744369, -5.231040848230092092E-16 ) ) ;
#6194=CYLINDRICAL_SURFACE ( 'NONE', #3749, 6.500000000000001776 ) ;
#6196=CARTESIAN_POINT ( 'NONE',  ( 14.38741851828413942, 8.077882666870964457, -2.999999999999992895 ) ) ;
#6206=LINE ( 'NONE', #922, #2558 ) ;
#6209=CARTESIAN_POINT ( 'NONE',  ( -40.82267254781529431, -94.88271315313488685, -9.511447951234663500E-14 ) ) ;
#6212=ORIENTED_EDGE ( 'NONE', *, *, #5562, .F. ) ;
#6220=ORIENTED_EDGE ( 'NONE', *, *, #786, .F. ) ;
#6226=DIRECTION ( 'NONE',  ( -5.715354789860003484E-18, -9.999836672264337477E-16, 1.000000000000000000 ) ) ;
#6234=ORIENTED_EDGE ( 'NONE', *, *, #6393, .T. ) ;
#6243=ORIENTED_EDGE ( 'NONE', *, *, #5599, .F. ) ;
#6249=ADVANCED_FACE ( 'NONE', ( #4967 ), #5467, .T. ) ;
#6256=CARTESIAN_POINT ( 'NONE',  ( -16.51707533432788111, -40.85914143033993895, -3.000000000000041744 ) ) ;
#6260=LINE ( 'NONE', #1621, #5898 ) ;
#6261=DIRECTION ( 'NONE',  ( 5.715354789860003484E-18, 9.999836672264337477E-16, -1.000000000000000000 ) ) ;
#6263=CIRCLE ( 'NONE', #7212, 147.0000000000000284 ) ;
#6270=ORIENTED_EDGE ( 'NONE', *, *, #1743, .F. ) ;
#6272=ADVANCED_FACE ( 'NONE', ( #3859 ), #5039, .F. ) ;
#6274=VECTOR ( 'NONE', #1861, 1000.000000000000000 ) ;
#6275=LINE ( 'NONE', #13, #5831 ) ;
#6279=DIRECTION ( 'NONE',  ( -0.9793199139485100346, -0.2023178344681531293, -1.787644449902631965E-16 ) ) ;
#6283=ORIENTED_EDGE ( 'NONE', *, *, #27, .F. ) ;
#6285=LINE ( 'NONE', #2843, #4367 ) ;
#6286=DIRECTION ( 'NONE',  ( -5.715354789860003484E-18, -9.999836672264337477E-16, 1.000000000000000000 ) ) ;
#6295=MECHANICAL_DESIGN_GEOMETRIC_PRESENTATION_REPRESENTATION('',(#5594),#4260);
#6298=CARTESIAN_POINT ( 'NONE',  ( -3.749938752099124972, 0.02143258046197846906, -3.000000000000000888 ) ) ;
#6300=FACE_OUTER_BOUND ( 'NONE', #1223, .T. ) ;
#6308=FACE_OUTER_BOUND ( 'NONE', #1863, .T. ) ;
#6309=AXIS2_PLACEMENT_3D ( 'NONE', #4655, #4, #4611 ) ;
#6310=CARTESIAN_POINT ( 'NONE',  ( -45.28625779897078729, -94.36209361619114588, -3.000000000000095479 ) ) ;
#6315=VECTOR ( 'NONE', #7193, 1000.000000000000000 ) ;
#6320=ORIENTED_EDGE ( 'NONE', *, *, #1650, .F. ) ;
#6323=VERTEX_POINT ( 'NONE', #3903 ) ;
#6325=ORIENTED_EDGE ( 'NONE', *, *, #1314, .T. ) ;
#6329=ADVANCED_FACE ( 'NONE', ( #4555 ), #2163, .T. ) ;
#6339=VERTEX_POINT ( 'NONE', #6177 ) ;
#6343=ADVANCED_FACE ( 'NONE', ( #2124 ), #3940, .F. ) ;
#6344=CARTESIAN_POINT ( 'NONE',  ( -45.28625779897078729, -94.36209361619114588, -3.000000000000095479 ) ) ;
#6347=VERTEX_POINT ( 'NONE', #5649 ) ;
#6349=( NAMED_UNIT ( * ) SI_UNIT ( $, .STERADIAN. ) SOLID_ANGLE_UNIT ( ) );
#6354=EDGE_LOOP ( 'NONE', ( #342, #1964, #1623, #6243 ) ) ;
#6363=ORIENTED_EDGE ( 'NONE', *, *, #5054, .T. ) ;
#6368=CARTESIAN_POINT ( 'NONE',  ( -32.93157973858376408, 14.54341967768581867, -2.999999999999986677 ) ) ;
#6375=DIRECTION ( 'NONE',  ( 5.715354789860003484E-18, 9.999836672264337477E-16, -1.000000000000000000 ) ) ;
#6377=ORIENTED_EDGE ( 'NONE', *, *, #4995, .T. ) ;
#6381=( LENGTH_UNIT ( ) NAMED_UNIT ( * ) SI_UNIT ( .MILLI., .METRE. ) );
#6386=DIRECTION ( 'NONE',  ( -5.715354789860003484E-18, -9.999836672264337477E-16, 1.000000000000000000 ) ) ;
#6389=ORIENTED_EDGE ( 'NONE', *, *, #4849, .T. ) ;
#6393=EDGE_CURVE ( 'NONE', #961, #4283, #6761, .T. ) ;
#6400=CARTESIAN_POINT ( 'NONE',  ( -28.22553731214382111, -35.79092421365019305, -3.001000000000037193 ) ) ;
#6410=CIRCLE ( 'NONE', #398, 2.500000000000000000 ) ;
#6421=CARTESIAN_POINT ( 'NONE',  ( -14.70408710852078116, -35.66654345889202204, -3.575000000000001175E-14 ) ) ;
#6427=DIRECTION ( 'NONE',  ( -0.2023178344681547114, 0.9793199139485095905, 8.673617379884032514E-16 ) ) ;
#6432=CARTESIAN_POINT ( 'NONE',  ( -15.80406914246985650, -35.66025656862317561, -3.000000000000036415 ) ) ;
#6433=CARTESIAN_POINT ( 'NONE',  ( -33.94153943842304955, 12.25650441806195445, 1.206231629534596424E-14 ) ) ;
#6436=ORIENTED_EDGE ( 'NONE', *, *, #4849, .F. ) ;
#6450=EDGE_CURVE ( 'NONE', #5997, #6064, #875, .T. ) ;
#6455=LINE ( 'NONE', #2312, #967 ) ;
#6458=ORIENTED_EDGE ( 'NONE', *, *, #3293, .T. ) ;
#6460=DIRECTION ( 'NONE',  ( 0.8795363392562568494, -0.4758317222797389667, -4.707970883985391064E-16 ) ) ;
#6461=ORIENTED_EDGE ( 'NONE', *, *, #1409, .T. ) ;
#6465=ORIENTED_EDGE ( 'NONE', *, *, #1153, .T. ) ;
#6467=DIRECTION ( 'NONE',  ( 1.000000000000000000, 0.000000000000000000, 0.000000000000000000 ) ) ;
#6469=CARTESIAN_POINT ( 'NONE',  ( 7.283874945971848369, -8.906884184084093548, -3.000000000000009770 ) ) ;
#6471=LINE ( 'NONE', #4784, #5661 ) ;
#6480=CIRCLE ( 'NONE', #7443, 0.7500000000000000000 ) ;
#6492=DIRECTION ( 'NONE',  ( 0.4039838799357178822, 0.9147661038495488173, -2.999999999999999208E-14 ) ) ;
#6503=DIRECTION ( 'NONE',  ( -5.715354789860003484E-18, -9.999836672264337477E-16, 1.000000000000000000 ) ) ;
#6507=ADVANCED_FACE ( 'NONE', ( #6995, #4603 ), #3493, .T. ) ;
#6515=ADVANCED_FACE ( 'NONE', ( #3038 ), #1840, .F. ) ;
#6521=CARTESIAN_POINT ( 'NONE',  ( -19.94212619460463287, -40.63668738334721553, -3.000000000000041744 ) ) ;
#6524=DIRECTION ( 'NONE',  ( 0.9793199139485104787, 0.2023178344681509366, 2.079116908177630447E-16 ) ) ;
#6525=CIRCLE ( 'NONE', #4374, 0.7500000000000000000 ) ;
#6529=VECTOR ( 'NONE', #5546, 1000.000000000000227 ) ;
#6551=PRESENTATION_STYLE_ASSIGNMENT (( #4078 ) ) ;
#6555=EDGE_CURVE ( 'NONE', #4778, #7025, #7253, .T. ) ;
#6560=ADVANCED_FACE ( 'NONE', ( #1979 ), #2051, .T. ) ;
#6562=CARTESIAN_POINT ( 'NONE',  ( -28.68093632328499965, 11.79168739492699913, -1.500000000001999956 ) ) ;
#6571=DIRECTION ( 'NONE',  ( 0.8056443796264692869, -0.5923994712829185882, -5.877852522924713037E-16 ) ) ;
#6581=ORIENTED_EDGE ( 'NONE', *, *, #6642, .T. ) ;
#6597=VERTEX_POINT ( 'NONE', #4290 ) ;
#6622=DIRECTION ( 'NONE',  ( 5.715354789860003484E-18, 9.999836672264337477E-16, -1.000000000000000000 ) ) ;
#6624=VERTEX_POINT ( 'NONE', #2480 ) ;
#6627=CARTESIAN_POINT ( 'NONE',  ( -33.94153943842304955, 12.25650441806195801, -2.999999999999988898 ) ) ;
#6628=EDGE_CURVE ( 'NONE', #716, #2186, #6075, .T. ) ;
#6636=ORIENTED_EDGE ( 'NONE', *, *, #668, .F. ) ;
#6637=DIRECTION ( 'NONE',  ( -0.9999836672264332815, 0.005715354789859876036, 0.000000000000000000 ) ) ;
#6638=CIRCLE ( 'NONE', #3395, 0.7499999999999893419 ) ;
#6642=EDGE_CURVE ( 'NONE', #3409, #1452, #4365, .T. ) ;
#6647=ORIENTED_EDGE ( 'NONE', *, *, #4805, .T. ) ;
#6651=VECTOR ( 'NONE', #5424, 999.9999999999998863 ) ;
#6665=AXIS2_PLACEMENT_3D ( 'NONE', #4383, #5521, #1139 ) ;
#6667=CARTESIAN_POINT ( 'NONE',  ( 10.02759472486470926, 5.630039434485818894, -2.999999999999995115 ) ) ;
#6678=VERTEX_POINT ( 'NONE', #5511 ) ;
#6679=VERTEX_POINT ( 'NONE', #334 ) ;
#6690=ORIENTED_EDGE ( 'NONE', *, *, #5399, .T. ) ;
#6692=DIRECTION ( 'NONE',  ( -5.715354789860003484E-18, -9.999836672264337477E-16, 1.000000000000000000 ) ) ;
#6699=ADVANCED_FACE ( 'NONE', ( #6032 ), #5342, .F. ) ;
#6700=ADVANCED_FACE ( 'NONE', ( #933 ), #3676, .F. ) ;
#6703=DIRECTION ( 'NONE',  ( 0.9147661038495488173, -0.4039838799357178822, 0.000000000000000000 ) ) ;
#6706=EDGE_CURVE ( 'NONE', #2728, #4894, #1134, .T. ) ;
#6718=ORIENTED_EDGE ( 'NONE', *, *, #419, .F. ) ;
#6724=DIRECTION ( 'NONE',  ( 0.9999836672264331705, -0.005715354789860001804, 0.000000000000000000 ) ) ;
#6725=FACE_OUTER_BOUND ( 'NONE', #696, .T. ) ;
#6729=CARTESIAN_POINT ( 'NONE',  ( -28.37794841333281681, 12.47776197281474708, -1.499999999999988010 ) ) ;
#6731=VECTOR ( 'NONE', #3392, 1000.000000000000000 ) ;
#6732=DIRECTION ( 'NONE',  ( -0.4758317222797389667, -0.8795363392562568494, -8.822415211014833627E-16 ) ) ;
#6735=DIRECTION ( 'NONE',  ( -5.715354789860003484E-18, -9.999836672264337477E-16, 1.000000000000000000 ) ) ;
#6748=DIRECTION ( 'NONE',  ( -0.06375834441969779887, -0.9979653668924884924, -9.983134689092966662E-16 ) ) ;
#6749=DIRECTION ( 'NONE',  ( -5.715354789860003484E-18, -9.999836672264337477E-16, 1.000000000000000000 ) ) ;
#6753=DIRECTION ( 'NONE',  ( -5.715354789860003484E-18, -9.999836672264337477E-16, 1.000000000000000000 ) ) ;
#6756=VERTEX_POINT ( 'NONE', #5078 ) ;
#6759=CARTESIAN_POINT ( 'NONE',  ( -44.78727511552453677, -94.39397278840091587, -3.001000000000095813 ) ) ;
#6761=LINE ( 'NONE', #3337, #2442 ) ;
#6773=AXIS2_PLACEMENT_3D ( 'NONE', #1152, #6971, #4719 ) ;
#6777=APPLICATION_CONTEXT ( 'automotive_design' ) ;
#6779=ADVANCED_FACE ( 'NONE', ( #6725 ), #2809, .T. ) ;
#6780=CARTESIAN_POINT ( 'NONE',  ( -17.04733905648494030, -8.234069079964157822, -3.000000000000009326 ) ) ;
#6782=DIRECTION ( 'NONE',  ( -0.9999836672264332815, 0.005715354789859876036, 0.000000000000000000 ) ) ;
#6785=LINE ( 'NONE', #6821, #2083 ) ;
#6798=ORIENTED_EDGE ( 'NONE', *, *, #619, .T. ) ;
#6800=ORIENTED_EDGE ( 'NONE', *, *, #4995, .F. ) ;
#6803=CARTESIAN_POINT ( 'NONE',  ( -32.93157973858376408, 14.54341967768581867, -2.999999999999986677 ) ) ;
#6807=ORIENTED_EDGE ( 'NONE', *, *, #5599, .T. ) ;
#6813=DIRECTION ( 'NONE',  ( 0.9979653668924883814, -0.06375834441969779887, -5.805357692931203648E-17 ) ) ;
#6814=ORIENTED_CLOSED_SHELL ( 'NONE', *, #3500, .F. );
#6815=ORIENTED_EDGE ( 'NONE', *, *, #1569, .T. ) ;
#6821=CARTESIAN_POINT ( 'NONE',  ( -32.93157973858376408, 14.54341967768581867, -2.999999999999986677 ) ) ;
#6825=DIRECTION ( 'NONE',  ( -0.9793199139485099236, -0.2023178344681531016, -1.787644449902631719E-16 ) ) ;
#6831=EDGE_CURVE ( 'NONE', #3341, #4778, #3257, .T. ) ;
#6833=ORIENTED_EDGE ( 'NONE', *, *, #1409, .F. ) ;
#6838=CARTESIAN_POINT ( 'NONE',  ( -35.54168210215662072, 14.82156649444486263, -2.250000000002000178 ) ) ;
#6851=CARTESIAN_POINT ( 'NONE',  ( -28.26642576027046516, -36.90973657692984489, -3.001000000000038082 ) ) ;
#6852=CARTESIAN_POINT ( 'NONE',  ( 37.98783301546301061, 6.414454976836671207, -1.055128867088878541 ) ) ;
#6855=CIRCLE ( 'NONE', #4094, 140.0000000000000284 ) ;
#6857=DIRECTION ( 'NONE',  ( -5.715354789860003484E-18, -9.999836672264337477E-16, 1.000000000000000000 ) ) ;
#6860=CARTESIAN_POINT ( 'NONE',  ( 37.86567095459282228, 7.005780695865149177, -1.500000000001998623 ) ) ;
#6861=EDGE_LOOP ( 'NONE', ( #2634, #6137, #6798, #6718 ) ) ;
#6884=ORIENTED_EDGE ( 'NONE', *, *, #2180, .F. ) ;
#6903=CARTESIAN_POINT ( 'NONE',  ( -40.65229780501022816, -93.90085982332443848, -9.413166846682193472E-14 ) ) ;
#6912=CARTESIAN_POINT ( 'NONE',  ( -40.82267254781529431, -94.88271315313488685, -3.000000000000095923 ) ) ;
#6920=ORIENTED_EDGE ( 'NONE', *, *, #910, .T. ) ;
#6923=LINE ( 'NONE', #5193, #4129 ) ;
#6930=DIRECTION ( 'NONE',  ( -5.715354789860003484E-18, -9.999836672264337477E-16, 1.000000000000000000 ) ) ;
#6934=ORIENTED_EDGE ( 'NONE', *, *, #4113, .F. ) ;
#6940=CARTESIAN_POINT ( 'NONE',  ( 104.0973215944787711, -119.5240462704291389, -3.000000000000119904 ) ) ;
#6941=CARTESIAN_POINT ( 'NONE',  ( -12.80424950550273167, -30.40040925781620373, -3.000000000000031086 ) ) ;
#6945=CARTESIAN_POINT ( 'NONE',  ( 1.714606436958001585E-17, 2.999951001679301835E-15, -3.000000000000000888 ) ) ;
#6971=DIRECTION ( 'NONE',  ( 5.715354789860003484E-18, 9.999836672264337477E-16, -1.000000000000000000 ) ) ;
#6980=LINE ( 'NONE', #664, #6274 ) ;
#6984=AXIS2_PLACEMENT_3D ( 'NONE', #171, #7125, #4345 ) ;
#6985=CARTESIAN_POINT ( 'NONE',  ( -12.36403222600316276, 10.92614786255227166, -2.999999999999990230 ) ) ;
#6990=VERTEX_POINT ( 'NONE', #1477 ) ;
#6992=VECTOR ( 'NONE', #2748, 1000.000000000000000 ) ;
#6994=CARTESIAN_POINT ( 'NONE',  ( -28.22553731214382111, -35.79092421365019305, -3.000000000000036859 ) ) ;
#6995=FACE_BOUND ( 'NONE', #5234, .T. ) ;
#6996=DIRECTION ( 'NONE',  ( -0.9858503002877112564, 0.1676281164441980331, 1.619908943762944784E-16 ) ) ;
#7004=CARTESIAN_POINT ( 'NONE',  ( -35.54168210215661361, 14.82156649444488394, -1.500000000001999956 ) ) ;
#7018=FACE_OUTER_BOUND ( 'NONE', #1974, .T. ) ;
#7019=CARTESIAN_POINT ( 'NONE',  ( -13.19674249314596892, -2.997380612392114951, -3.072755722272031268E-15 ) ) ;
#7021=EDGE_LOOP ( 'NONE', ( #1119, #2875, #3833, #7147 ) ) ;
#7022=EDGE_CURVE ( 'NONE', #6347, #2788, #3045, .T. ) ;
#7024=ORIENTED_EDGE ( 'NONE', *, *, #5487, .T. ) ;
#7025=VERTEX_POINT ( 'NONE', #2680 ) ;
#7035=( NAMED_UNIT ( * ) PLANE_ANGLE_UNIT ( ) SI_UNIT ( $, .RADIAN. ) );
#7036=CARTESIAN_POINT ( 'NONE',  ( -45.21893524706405287, -93.36435596057614816, -3.001000000000094925 ) ) ;
#7050=DIRECTION ( 'NONE',  ( 0.9123165276958903336, 0.4094857180573137079, 4.146932426562371539E-16 ) ) ;
#7056=VERTEX_POINT ( 'NONE', #7231 ) ;
#7057=ORIENTED_EDGE ( 'NONE', *, *, #3831, .T. ) ;
#7058=EDGE_LOOP ( 'NONE', ( #22, #3697, #1385, #7066 ) ) ;
#7062=ADVANCED_FACE ( 'NONE', ( #3648 ), #4866, .F. ) ;
#7065=DIRECTION ( 'NONE',  ( 5.715354789860003484E-18, 9.999836672264337477E-16, -1.000000000000000000 ) ) ;
#7066=ORIENTED_EDGE ( 'NONE', *, *, #1040, .F. ) ;
#7069=CARTESIAN_POINT ( 'NONE',  ( -28.68093632328457332, 11.79168739492758711, -1.499999999999988676 ) ) ;
#7070=CARTESIAN_POINT ( 'NONE',  ( -14.70408710852078116, -35.66654345889202204, -3.000000000000036415 ) ) ;
#7071=DIRECTION ( 'NONE',  ( -0.9147661038495488173, 0.4039838799357178822, 1.577721810442023611E-30 ) ) ;
#7078=DIRECTION ( 'NONE',  ( 0.8474369140690223290, -0.5308961072311347840, -5.260440335992994916E-16 ) ) ;
#7080=CARTESIAN_POINT ( 'NONE',  ( 94.42889356597736139, -103.2882618349535591, -3.000000000000103917 ) ) ;
#7085=LINE ( 'NONE', #874, #1339 ) ;
#7087=VERTEX_POINT ( 'NONE', #787 ) ;
#7092=ORIENTED_EDGE ( 'NONE', *, *, #3471, .T. ) ;
#7094=EDGE_LOOP ( 'NONE', ( #1981, #6084, #7436, #6690, #4398, #4738, #1440, #6054, #852, #5145, #3554, #1530, #6088, #5237, #6363, #6581, #182, #1352, #1674, #2024, #7128, #2422, #6320, #4031, #4399, #5385, #2700, #4928, #405, #2984 ) ) ;
#7097=DIRECTION ( 'NONE',  ( -0.9147661038495495944, 0.4039838799357160504, 3.987490689252424829E-16 ) ) ;
#7103=CIRCLE ( 'NONE', #3857, 1.100000000000000755 ) ;
#7105=DIRECTION ( 'NONE',  ( 0.9999836672264332815, -0.005715354789859936752, 0.000000000000000000 ) ) ;
#7109=VECTOR ( 'NONE', #4443, 999.9999999999998863 ) ;
#7118=CYLINDRICAL_SURFACE ( 'NONE', #6083, 140.0000000000000284 ) ;
#7125=DIRECTION ( 'NONE',  ( -5.715354789860004255E-18, -9.999836672264337477E-16, 1.000000000000000000 ) ) ;
#7128=ORIENTED_EDGE ( 'NONE', *, *, #526, .T. ) ;
#7129=VECTOR ( 'NONE', #7194, 1000.000000000000000 ) ;
#7131=CARTESIAN_POINT ( 'NONE',  ( -35.54168210215662072, 14.82156649444486263, -2.250000000002000178 ) ) ;
#7132=AXIS2_PLACEMENT_3D ( 'NONE', #4594, #2248, #524 ) ;
#7145=ADVANCED_FACE ( 'NONE', ( #613 ), #4620, .F. ) ;
#7147=ORIENTED_EDGE ( 'NONE', *, *, #112, .T. ) ;
#7154=ORIENTED_EDGE ( 'NONE', *, *, #1362, .F. ) ;
#7157=DIRECTION ( 'NONE',  ( 0.9999836672264331705, -0.005715354789860049509, 0.000000000000000000 ) ) ;
#7162=ORIENTED_EDGE ( 'NONE', *, *, #5139, .F. ) ;
#7163=VERTEX_POINT ( 'NONE', #5261 ) ;
#7175=BREP_WITH_VOIDS ( 'NONE', #5921, ( #6814, #925 ) );
#7179=CARTESIAN_POINT ( 'NONE',  ( -15.52817266570582611, -38.02681526409561741, -3.000000000000039080 ) ) ;
#7182=VERTEX_POINT ( 'NONE', #5428 ) ;
#7183=EDGE_CURVE ( 'NONE', #4278, #1742, #2169, .T. ) ;
#7184=CARTESIAN_POINT ( 'NONE',  ( -28.98392423323678813, 11.10561281703983738, -1.499999999999988676 ) ) ;
#7191=EDGE_CURVE ( 'NONE', #5220, #815, #422, .T. ) ;
#7193=DIRECTION ( 'NONE',  ( -5.715354789860003484E-18, -9.999836672264337477E-16, 1.000000000000000000 ) ) ;
#7194=DIRECTION ( 'NONE',  ( -5.715354789860003484E-18, -9.999836672264337477E-16, 1.000000000000000000 ) ) ;
#7202=ADVANCED_FACE ( 'NONE', ( #1578 ), #4483, .F. ) ;
#7203=CARTESIAN_POINT ( 'NONE',  ( 14.38741851828413942, 8.077882666870960904, 8.159979933984663174E-15 ) ) ;
#7204=AXIS2_PLACEMENT_3D ( 'NONE', #3383, #5698, #535 ) ;
#7210=ORIENTED_EDGE ( 'NONE', *, *, #5562, .T. ) ;
#7212=AXIS2_PLACEMENT_3D ( 'NONE', #3952, #6261, #7414 ) ;
#7216=VECTOR ( 'NONE', #5722, 999.9999999999998863 ) ;
#7219=EDGE_LOOP ( 'NONE', ( #5841, #5199, #5904, #2477, #6934, #6833, #5321, #2585, #2913, #6884, #1107, #1584, #3916, #5669, #6800, #814, #4689, #6212, #2952, #2543, #6146, #5118, #4574, #1871, #5793, #6270, #1459, #1649, #3019, #2552 ) ) ;
#7225=CARTESIAN_POINT ( 'NONE',  ( -40.82267254781525168, -94.88271315313488685, -3.000000000000095923 ) ) ;
#7230=DIRECTION ( 'NONE',  ( 0.9993328523369457983, -0.03652191451860404420, -3.080977621017558246E-17 ) ) ;
#7231=CARTESIAN_POINT ( 'NONE',  ( -3.749938752099124972, 0.02143258046197547145, 4.592425496802572929E-31 ) ) ;
#7241=VECTOR ( 'NONE', #5343, 1000.000000000000000 ) ;
#7242=DIRECTION ( 'NONE',  ( -0.8043765792067081311, 0.5941197849118596830, 5.895127837531212072E-16 ) ) ;
#7253=CIRCLE ( 'NONE', #2205, 2.999999999999999556 ) ;
#7255=CARTESIAN_POINT ( 'NONE',  ( 3.749938752099124972, -0.02143258046197501002, 0.000000000000000000 ) ) ;
#7256=CARTESIAN_POINT ( 'NONE',  ( 15.39900769062488806, 3.181283097128406290, -2.999999999999997335 ) ) ;
#7264=DIRECTION ( 'NONE',  ( -0.9793199139485099236, -0.2023178344681531016, -1.787644449902631719E-16 ) ) ;
#7266=VERTEX_POINT ( 'NONE', #7184 ) ;
#7271=CARTESIAN_POINT ( 'NONE',  ( 0.000000000000000000, 0.000000000000000000, 0.000000000000000000 ) ) ;
#7280=EDGE_LOOP ( 'NONE', ( #563, #2275, #5171, #4196 ) ) ;
#7291=ORIENTED_EDGE ( 'NONE', *, *, #4197, .T. ) ;
#7292=VERTEX_POINT ( 'NONE', #2018 ) ;
#7310=DIRECTION ( 'NONE',  ( 0.9123165276958903336, 0.4094857180573137079, 4.146932426562371539E-16 ) ) ;
#7319=AXIS2_PLACEMENT_3D ( 'NONE', #4870, #308, #3229 ) ;
#7337=AXIS2_PLACEMENT_3D ( 'NONE', #4193, #6386, #5838 ) ;
#7338=EDGE_LOOP ( 'NONE', ( #5990, #2054, #7210, #4698 ) ) ;
#7339=FACE_OUTER_BOUND ( 'NONE', #6861, .T. ) ;
#7340=CARTESIAN_POINT ( 'NONE',  ( -19.94212619460463287, -40.63668738334721553, -3.001000000000041634 ) ) ;
#7344=ORIENTED_EDGE ( 'NONE', *, *, #5477, .F. ) ;
#7347=DIRECTION ( 'NONE',  ( 9.251858538542970644E-15, 2.775557561562891351E-14, 1.000000000000000000 ) ) ;
#7354=ORIENTED_EDGE ( 'NONE', *, *, #6628, .T. ) ;
#7362=CARTESIAN_POINT ( 'NONE',  ( -28.26642576027046516, -36.90973657692984489, -3.001000000000038082 ) ) ;
#7381=CARTESIAN_POINT ( 'NONE',  ( -33.25476684253234794, 13.81160679460617757, -1.499999999999986899 ) ) ;
#7392=ADVANCED_FACE ( 'NONE', ( #1056 ), #2216, .T. ) ;
#7396=CYLINDRICAL_SURFACE ( 'NONE', #1330, 0.7499999999999994449 ) ;
#7398=ORIENTED_EDGE ( 'NONE', *, *, #619, .F. ) ;
#7401=DIRECTION ( 'NONE',  ( -5.715354789860003484E-18, -9.999836672264337477E-16, 1.000000000000000000 ) ) ;
#7411=DIRECTION ( 'NONE',  ( 0.9999836672264332815, -0.005715354789859183882, 0.000000000000000000 ) ) ;
#7412=CARTESIAN_POINT ( 'NONE',  ( -33.25476684253263215, 13.81160679460551677, -2.250000000002000178 ) ) ;
#7414=DIRECTION ( 'NONE',  ( -0.9999836672264332815, 0.005715354789859956701, 0.000000000000000000 ) ) ;
#7418=PLANE ( 'NONE',  #1734 ) ;
#7423=EDGE_CURVE ( 'NONE', #577, #937, #1618, .T. ) ;
#7429=LINE ( 'NONE', #3442, #3636 ) ;
#7430=CARTESIAN_POINT ( 'NONE',  ( -32.93157973858376408, 14.54341967768581512, 1.435496648130876646E-14 ) ) ;
#7436=ORIENTED_EDGE ( 'NONE', *, *, #1631, .T. ) ;
#7441=ORIENTED_EDGE ( 'NONE', *, *, #2504, .T. ) ;
#7442=VERTEX_POINT ( 'NONE', #3489 ) ;
#7443=AXIS2_PLACEMENT_3D ( 'NONE', #7004, #752, #194 ) ;
#7444=DIRECTION ( 'NONE',  ( -0.03652191451860400950, -0.9993328523369456873, -9.995252661588299226E-16 ) ) ;
ENDSEC;
END-ISO-10303-21;
